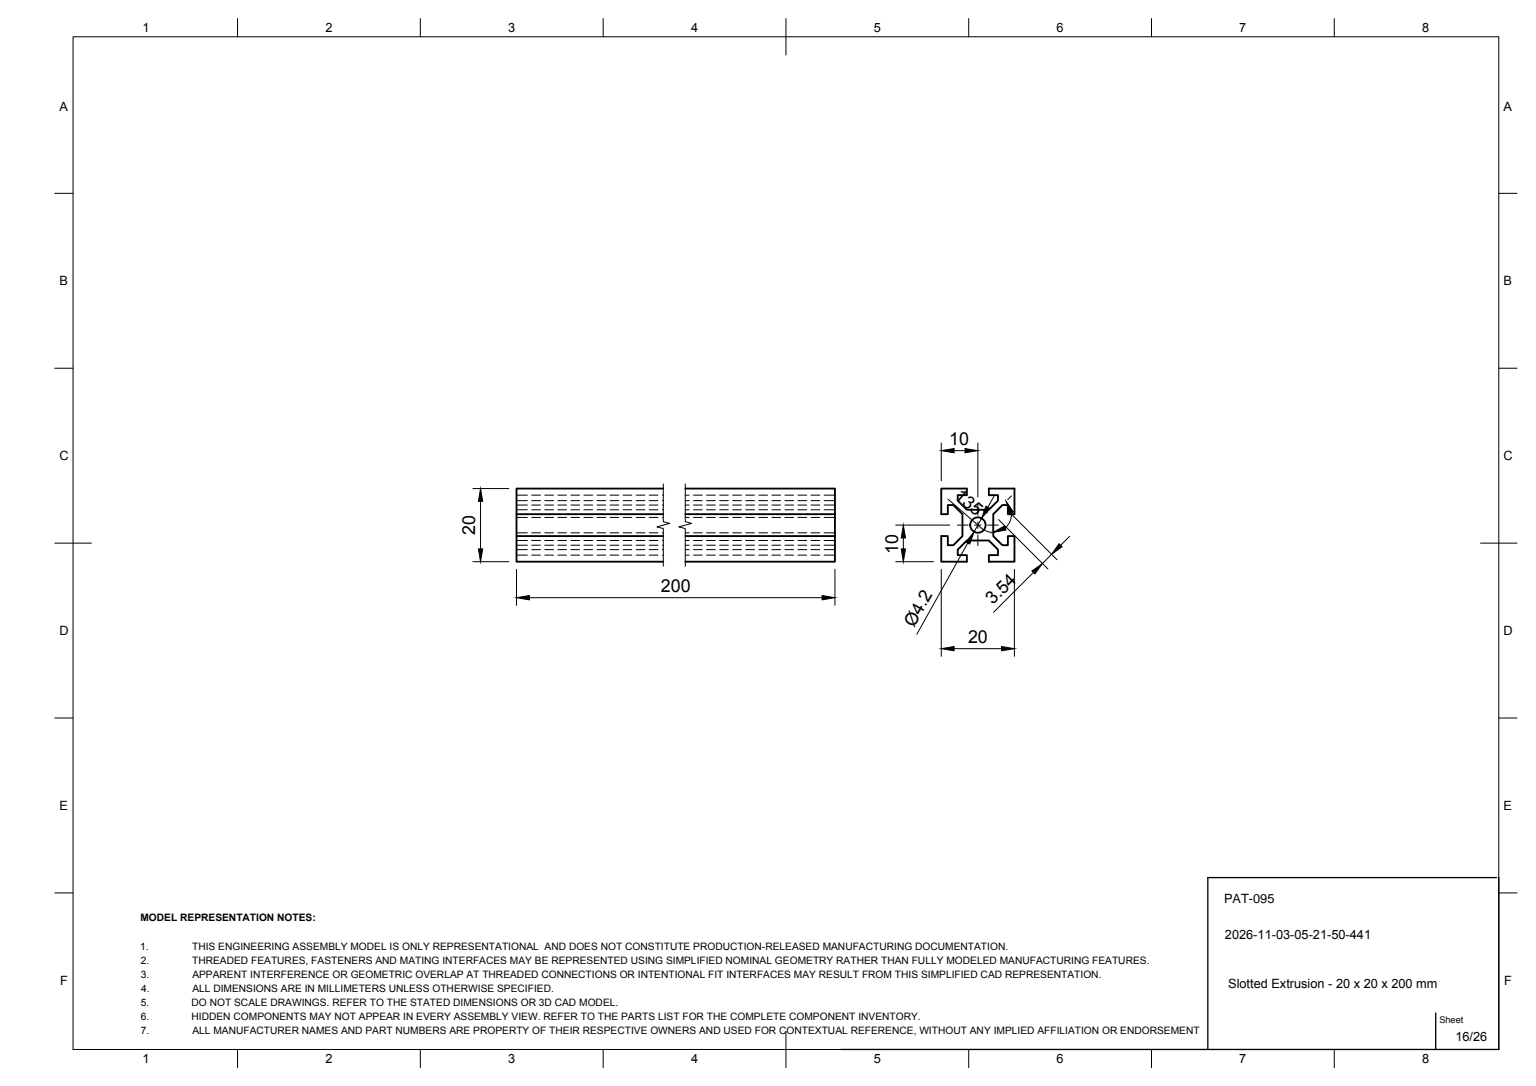
ISO-10303-21;
HEADER;
/* Generated by software containing ST-Developer
 * from STEP Tools, Inc. (www.steptools.com) 
 */

FILE_DESCRIPTION(
/* description */ ('Single-Axis Profile-Rail Linear Slide'),
/* implementation_level */ '2;1');

FILE_NAME(
/* name */ 'Slotted Extrusion - 20 x 20 x 200 mm.step',
/* time_stamp */ '2026-10-27T10:47:43-07:00',
/* author */ (''),
/* organization */ (''),
/* preprocessor_version */ 'ST-DEVELOPER v20.2',
/* originating_system */ 'Autodesk Translation Framework v15.17.0.0',
/* authorisation */ '');

FILE_SCHEMA (('AUTOMOTIVE_DESIGN { 1 0 10303 214 3 1 1 }'));
ENDSEC;

DATA;
#10=MECHANICAL_DESIGN_GEOMETRIC_PRESENTATION_REPRESENTATION('',(#340),#14478);
#286=SHAPE_REPRESENTATION_RELATIONSHIP('SRR','None',#14616,#313);
#313=ADVANCED_BREP_SHAPE_REPRESENTATION('',(#367),#14460);
#340=STYLED_ITEM('',(#14845),#367);
#367=MANIFOLD_SOLID_BREP('Body1',#8600);
#434=FACE_BOUND('',#1627,.T.);
#435=FACE_BOUND('',#1629,.T.);
#666=PLANE('',#9227);
#667=PLANE('',#9228);
#668=PLANE('',#9229);
#669=PLANE('',#9230);
#670=PLANE('',#9231);
#671=PLANE('',#9232);
#672=PLANE('',#9233);
#673=PLANE('',#9234);
#674=PLANE('',#9235);
#675=PLANE('',#9236);
#676=PLANE('',#9237);
#677=PLANE('',#9238);
#678=PLANE('',#9239);
#679=PLANE('',#9240);
#680=PLANE('',#9241);
#681=PLANE('',#9242);
#682=PLANE('',#9243);
#683=PLANE('',#9244);
#684=PLANE('',#9245);
#685=PLANE('',#9246);
#686=PLANE('',#9247);
#687=PLANE('',#9248);
#688=PLANE('',#9249);
#689=PLANE('',#9250);
#690=PLANE('',#9251);
#691=PLANE('',#9252);
#692=PLANE('',#9253);
#693=PLANE('',#9254);
#694=PLANE('',#9255);
#695=PLANE('',#9256);
#696=PLANE('',#9257);
#697=PLANE('',#9258);
#698=PLANE('',#9259);
#699=PLANE('',#9260);
#700=PLANE('',#9261);
#701=PLANE('',#9262);
#702=PLANE('',#9266);
#703=PLANE('',#9267);
#704=PLANE('',#9268);
#705=PLANE('',#9269);
#706=PLANE('',#9270);
#707=PLANE('',#9271);
#708=PLANE('',#9272);
#709=PLANE('',#9273);
#710=PLANE('',#9274);
#711=PLANE('',#9275);
#1070=FACE_OUTER_BOUND('',#1581,.T.);
#1071=FACE_OUTER_BOUND('',#1582,.T.);
#1072=FACE_OUTER_BOUND('',#1583,.T.);
#1073=FACE_OUTER_BOUND('',#1584,.T.);
#1074=FACE_OUTER_BOUND('',#1585,.T.);
#1075=FACE_OUTER_BOUND('',#1586,.T.);
#1076=FACE_OUTER_BOUND('',#1587,.T.);
#1077=FACE_OUTER_BOUND('',#1588,.T.);
#1078=FACE_OUTER_BOUND('',#1589,.T.);
#1079=FACE_OUTER_BOUND('',#1590,.T.);
#1080=FACE_OUTER_BOUND('',#1591,.T.);
#1081=FACE_OUTER_BOUND('',#1592,.T.);
#1082=FACE_OUTER_BOUND('',#1593,.T.);
#1083=FACE_OUTER_BOUND('',#1594,.T.);
#1084=FACE_OUTER_BOUND('',#1595,.T.);
#1085=FACE_OUTER_BOUND('',#1596,.T.);
#1086=FACE_OUTER_BOUND('',#1597,.T.);
#1087=FACE_OUTER_BOUND('',#1598,.T.);
#1088=FACE_OUTER_BOUND('',#1599,.T.);
#1089=FACE_OUTER_BOUND('',#1600,.T.);
#1090=FACE_OUTER_BOUND('',#1601,.T.);
#1091=FACE_OUTER_BOUND('',#1602,.T.);
#1092=FACE_OUTER_BOUND('',#1603,.T.);
#1093=FACE_OUTER_BOUND('',#1604,.T.);
#1094=FACE_OUTER_BOUND('',#1605,.T.);
#1095=FACE_OUTER_BOUND('',#1606,.T.);
#1096=FACE_OUTER_BOUND('',#1607,.T.);
#1097=FACE_OUTER_BOUND('',#1608,.T.);
#1098=FACE_OUTER_BOUND('',#1609,.T.);
#1099=FACE_OUTER_BOUND('',#1610,.T.);
#1100=FACE_OUTER_BOUND('',#1611,.T.);
#1101=FACE_OUTER_BOUND('',#1612,.T.);
#1102=FACE_OUTER_BOUND('',#1613,.T.);
#1103=FACE_OUTER_BOUND('',#1614,.T.);
#1104=FACE_OUTER_BOUND('',#1615,.T.);
#1105=FACE_OUTER_BOUND('',#1616,.T.);
#1106=FACE_OUTER_BOUND('',#1617,.T.);
#1107=FACE_OUTER_BOUND('',#1618,.T.);
#1108=FACE_OUTER_BOUND('',#1619,.T.);
#1109=FACE_OUTER_BOUND('',#1620,.T.);
#1110=FACE_OUTER_BOUND('',#1621,.T.);
#1111=FACE_OUTER_BOUND('',#1622,.T.);
#1112=FACE_OUTER_BOUND('',#1623,.T.);
#1113=FACE_OUTER_BOUND('',#1624,.T.);
#1114=FACE_OUTER_BOUND('',#1625,.T.);
#1115=FACE_OUTER_BOUND('',#1626,.T.);
#1116=FACE_OUTER_BOUND('',#1628,.T.);
#1581=EDGE_LOOP('',(#7013,#7014,#7015,#7016));
#1582=EDGE_LOOP('',(#7017,#7018,#7019,#7020));
#1583=EDGE_LOOP('',(#7021,#7022,#7023,#7024));
#1584=EDGE_LOOP('',(#7025,#7026,#7027,#7028));
#1585=EDGE_LOOP('',(#7029,#7030,#7031,#7032));
#1586=EDGE_LOOP('',(#7033,#7034,#7035,#7036));
#1587=EDGE_LOOP('',(#7037,#7038,#7039,#7040));
#1588=EDGE_LOOP('',(#7041,#7042,#7043,#7044));
#1589=EDGE_LOOP('',(#7045,#7046,#7047,#7048));
#1590=EDGE_LOOP('',(#7049,#7050,#7051,#7052));
#1591=EDGE_LOOP('',(#7053,#7054,#7055,#7056));
#1592=EDGE_LOOP('',(#7057,#7058,#7059,#7060));
#1593=EDGE_LOOP('',(#7061,#7062,#7063,#7064));
#1594=EDGE_LOOP('',(#7065,#7066,#7067,#7068));
#1595=EDGE_LOOP('',(#7069,#7070,#7071,#7072));
#1596=EDGE_LOOP('',(#7073,#7074,#7075,#7076));
#1597=EDGE_LOOP('',(#7077,#7078,#7079,#7080));
#1598=EDGE_LOOP('',(#7081,#7082,#7083,#7084));
#1599=EDGE_LOOP('',(#7085,#7086,#7087,#7088));
#1600=EDGE_LOOP('',(#7089,#7090,#7091,#7092));
#1601=EDGE_LOOP('',(#7093,#7094,#7095,#7096));
#1602=EDGE_LOOP('',(#7097,#7098,#7099,#7100));
#1603=EDGE_LOOP('',(#7101,#7102,#7103,#7104));
#1604=EDGE_LOOP('',(#7105,#7106,#7107,#7108));
#1605=EDGE_LOOP('',(#7109,#7110,#7111,#7112));
#1606=EDGE_LOOP('',(#7113,#7114,#7115,#7116));
#1607=EDGE_LOOP('',(#7117,#7118,#7119,#7120));
#1608=EDGE_LOOP('',(#7121,#7122,#7123,#7124));
#1609=EDGE_LOOP('',(#7125,#7126,#7127,#7128));
#1610=EDGE_LOOP('',(#7129,#7130,#7131,#7132));
#1611=EDGE_LOOP('',(#7133,#7134,#7135,#7136));
#1612=EDGE_LOOP('',(#7137,#7138,#7139,#7140));
#1613=EDGE_LOOP('',(#7141,#7142,#7143,#7144));
#1614=EDGE_LOOP('',(#7145,#7146,#7147,#7148));
#1615=EDGE_LOOP('',(#7149,#7150,#7151,#7152));
#1616=EDGE_LOOP('',(#7153,#7154,#7155,#7156));
#1617=EDGE_LOOP('',(#7157,#7158,#7159,#7160));
#1618=EDGE_LOOP('',(#7161,#7162,#7163,#7164));
#1619=EDGE_LOOP('',(#7165,#7166,#7167,#7168));
#1620=EDGE_LOOP('',(#7169,#7170,#7171,#7172));
#1621=EDGE_LOOP('',(#7173,#7174,#7175,#7176));
#1622=EDGE_LOOP('',(#7177,#7178,#7179,#7180));
#1623=EDGE_LOOP('',(#7181,#7182,#7183,#7184));
#1624=EDGE_LOOP('',(#7185,#7186,#7187,#7188));
#1625=EDGE_LOOP('',(#7189,#7190,#7191,#7192));
#1626=EDGE_LOOP('',(#7193,#7194,#7195,#7196,#7197,#7198,#7199,#7200,#7201,
#7202,#7203,#7204,#7205,#7206,#7207,#7208,#7209,#7210,#7211,#7212,#7213,
#7214,#7215,#7216,#7217,#7218,#7219,#7220,#7221,#7222,#7223,#7224,#7225,
#7226,#7227,#7228,#7229,#7230,#7231,#7232,#7233,#7234,#7235,#7236));
#1627=EDGE_LOOP('',(#7237));
#1628=EDGE_LOOP('',(#7238,#7239,#7240,#7241,#7242,#7243,#7244,#7245,#7246,
#7247,#7248,#7249,#7250,#7251,#7252,#7253,#7254,#7255,#7256,#7257,#7258,
#7259,#7260,#7261,#7262,#7263,#7264,#7265,#7266,#7267,#7268,#7269,#7270,
#7271,#7272,#7273,#7274,#7275,#7276,#7277,#7278,#7279,#7280,#7281));
#1629=EDGE_LOOP('',(#7282));
#2376=LINE('',#13243,#3347);
#2377=LINE('',#13245,#3348);
#2378=LINE('',#13247,#3349);
#2379=LINE('',#13248,#3350);
#2380=LINE('',#13251,#3351);
#2381=LINE('',#13253,#3352);
#2382=LINE('',#13254,#3353);
#2383=LINE('',#13257,#3354);
#2384=LINE('',#13259,#3355);
#2385=LINE('',#13260,#3356);
#2386=LINE('',#13263,#3357);
#2387=LINE('',#13265,#3358);
#2388=LINE('',#13266,#3359);
#2389=LINE('',#13269,#3360);
#2390=LINE('',#13271,#3361);
#2391=LINE('',#13272,#3362);
#2392=LINE('',#13275,#3363);
#2393=LINE('',#13277,#3364);
#2394=LINE('',#13278,#3365);
#2395=LINE('',#13281,#3366);
#2396=LINE('',#13283,#3367);
#2397=LINE('',#13284,#3368);
#2398=LINE('',#13287,#3369);
#2399=LINE('',#13289,#3370);
#2400=LINE('',#13290,#3371);
#2401=LINE('',#13293,#3372);
#2402=LINE('',#13295,#3373);
#2403=LINE('',#13296,#3374);
#2404=LINE('',#13300,#3375);
#2405=LINE('',#13302,#3376);
#2406=LINE('',#13304,#3377);
#2407=LINE('',#13305,#3378);
#2408=LINE('',#13308,#3379);
#2409=LINE('',#13310,#3380);
#2410=LINE('',#13311,#3381);
#2411=LINE('',#13314,#3382);
#2412=LINE('',#13316,#3383);
#2413=LINE('',#13317,#3384);
#2414=LINE('',#13320,#3385);
#2415=LINE('',#13322,#3386);
#2416=LINE('',#13323,#3387);
#2417=LINE('',#13326,#3388);
#2418=LINE('',#13328,#3389);
#2419=LINE('',#13329,#3390);
#2420=LINE('',#13332,#3391);
#2421=LINE('',#13334,#3392);
#2422=LINE('',#13335,#3393);
#2423=LINE('',#13338,#3394);
#2424=LINE('',#13340,#3395);
#2425=LINE('',#13341,#3396);
#2426=LINE('',#13344,#3397);
#2427=LINE('',#13346,#3398);
#2428=LINE('',#13347,#3399);
#2429=LINE('',#13350,#3400);
#2430=LINE('',#13352,#3401);
#2431=LINE('',#13353,#3402);
#2432=LINE('',#13357,#3403);
#2433=LINE('',#13359,#3404);
#2434=LINE('',#13361,#3405);
#2435=LINE('',#13362,#3406);
#2436=LINE('',#13365,#3407);
#2437=LINE('',#13367,#3408);
#2438=LINE('',#13368,#3409);
#2439=LINE('',#13371,#3410);
#2440=LINE('',#13373,#3411);
#2441=LINE('',#13374,#3412);
#2442=LINE('',#13377,#3413);
#2443=LINE('',#13379,#3414);
#2444=LINE('',#13380,#3415);
#2445=LINE('',#13383,#3416);
#2446=LINE('',#13385,#3417);
#2447=LINE('',#13386,#3418);
#2448=LINE('',#13389,#3419);
#2449=LINE('',#13391,#3420);
#2450=LINE('',#13392,#3421);
#2451=LINE('',#13395,#3422);
#2452=LINE('',#13397,#3423);
#2453=LINE('',#13398,#3424);
#2454=LINE('',#13401,#3425);
#2455=LINE('',#13403,#3426);
#2456=LINE('',#13404,#3427);
#2457=LINE('',#13407,#3428);
#2458=LINE('',#13409,#3429);
#2459=LINE('',#13410,#3430);
#2460=LINE('',#13414,#3431);
#2461=LINE('',#13416,#3432);
#2462=LINE('',#13418,#3433);
#2463=LINE('',#13419,#3434);
#2464=LINE('',#13422,#3435);
#2465=LINE('',#13424,#3436);
#2466=LINE('',#13425,#3437);
#2467=LINE('',#13428,#3438);
#2468=LINE('',#13430,#3439);
#2469=LINE('',#13431,#3440);
#2470=LINE('',#13434,#3441);
#2471=LINE('',#13436,#3442);
#2472=LINE('',#13437,#3443);
#2473=LINE('',#13440,#3444);
#2474=LINE('',#13442,#3445);
#2475=LINE('',#13443,#3446);
#2476=LINE('',#13446,#3447);
#2477=LINE('',#13448,#3448);
#2478=LINE('',#13449,#3449);
#2479=LINE('',#13452,#3450);
#2480=LINE('',#13454,#3451);
#2481=LINE('',#13455,#3452);
#2482=LINE('',#13458,#3453);
#2483=LINE('',#13460,#3454);
#2484=LINE('',#13461,#3455);
#2485=LINE('',#13464,#3456);
#2486=LINE('',#13466,#3457);
#2487=LINE('',#13467,#3458);
#2488=LINE('',#13472,#3459);
#2489=LINE('',#13476,#3460);
#2490=LINE('',#13478,#3461);
#2491=LINE('',#13479,#3462);
#2492=LINE('',#13482,#3463);
#2493=LINE('',#13484,#3464);
#2494=LINE('',#13485,#3465);
#2495=LINE('',#13487,#3466);
#2496=LINE('',#13488,#3467);
#2497=LINE('',#13491,#3468);
#2498=LINE('',#13493,#3469);
#2499=LINE('',#13494,#3470);
#2500=LINE('',#13496,#3471);
#2501=LINE('',#13497,#3472);
#2502=LINE('',#13500,#3473);
#2503=LINE('',#13502,#3474);
#2504=LINE('',#13503,#3475);
#2505=LINE('',#13505,#3476);
#2506=LINE('',#13506,#3477);
#2507=LINE('',#13508,#3478);
#2508=LINE('',#13509,#3479);
#3347=VECTOR('',#10775,1.);
#3348=VECTOR('',#10776,1.);
#3349=VECTOR('',#10777,1.);
#3350=VECTOR('',#10778,1.);
#3351=VECTOR('',#10781,1.);
#3352=VECTOR('',#10782,1.);
#3353=VECTOR('',#10783,1.);
#3354=VECTOR('',#10786,1.);
#3355=VECTOR('',#10787,1.);
#3356=VECTOR('',#10788,1.);
#3357=VECTOR('',#10791,1.);
#3358=VECTOR('',#10792,1.);
#3359=VECTOR('',#10793,1.);
#3360=VECTOR('',#10796,1.);
#3361=VECTOR('',#10797,1.);
#3362=VECTOR('',#10798,1.);
#3363=VECTOR('',#10801,1.);
#3364=VECTOR('',#10802,1.);
#3365=VECTOR('',#10803,1.);
#3366=VECTOR('',#10806,1.);
#3367=VECTOR('',#10807,1.);
#3368=VECTOR('',#10808,1.);
#3369=VECTOR('',#10811,1.);
#3370=VECTOR('',#10812,1.);
#3371=VECTOR('',#10813,1.);
#3372=VECTOR('',#10816,1.);
#3373=VECTOR('',#10817,1.);
#3374=VECTOR('',#10818,1.);
#3375=VECTOR('',#10821,1.);
#3376=VECTOR('',#10822,1.);
#3377=VECTOR('',#10823,1.);
#3378=VECTOR('',#10824,1.);
#3379=VECTOR('',#10827,1.);
#3380=VECTOR('',#10828,1.);
#3381=VECTOR('',#10829,1.);
#3382=VECTOR('',#10832,1.);
#3383=VECTOR('',#10833,1.);
#3384=VECTOR('',#10834,1.);
#3385=VECTOR('',#10837,1.);
#3386=VECTOR('',#10838,1.);
#3387=VECTOR('',#10839,1.);
#3388=VECTOR('',#10842,1.);
#3389=VECTOR('',#10843,1.);
#3390=VECTOR('',#10844,1.);
#3391=VECTOR('',#10847,1.);
#3392=VECTOR('',#10848,1.);
#3393=VECTOR('',#10849,1.);
#3394=VECTOR('',#10852,1.);
#3395=VECTOR('',#10853,1.);
#3396=VECTOR('',#10854,1.);
#3397=VECTOR('',#10857,1.);
#3398=VECTOR('',#10858,1.);
#3399=VECTOR('',#10859,1.);
#3400=VECTOR('',#10862,1.);
#3401=VECTOR('',#10863,1.);
#3402=VECTOR('',#10864,1.);
#3403=VECTOR('',#10867,1.);
#3404=VECTOR('',#10868,1.);
#3405=VECTOR('',#10869,1.);
#3406=VECTOR('',#10870,1.);
#3407=VECTOR('',#10873,1.);
#3408=VECTOR('',#10874,1.);
#3409=VECTOR('',#10875,1.);
#3410=VECTOR('',#10878,1.);
#3411=VECTOR('',#10879,1.);
#3412=VECTOR('',#10880,1.);
#3413=VECTOR('',#10883,1.);
#3414=VECTOR('',#10884,1.);
#3415=VECTOR('',#10885,1.);
#3416=VECTOR('',#10888,1.);
#3417=VECTOR('',#10889,1.);
#3418=VECTOR('',#10890,1.);
#3419=VECTOR('',#10893,1.);
#3420=VECTOR('',#10894,1.);
#3421=VECTOR('',#10895,1.);
#3422=VECTOR('',#10898,1.);
#3423=VECTOR('',#10899,1.);
#3424=VECTOR('',#10900,1.);
#3425=VECTOR('',#10903,1.);
#3426=VECTOR('',#10904,1.);
#3427=VECTOR('',#10905,1.);
#3428=VECTOR('',#10908,1.);
#3429=VECTOR('',#10909,1.);
#3430=VECTOR('',#10910,1.);
#3431=VECTOR('',#10913,1.);
#3432=VECTOR('',#10914,1.);
#3433=VECTOR('',#10915,1.);
#3434=VECTOR('',#10916,1.);
#3435=VECTOR('',#10919,1.);
#3436=VECTOR('',#10920,1.);
#3437=VECTOR('',#10921,1.);
#3438=VECTOR('',#10924,1.);
#3439=VECTOR('',#10925,1.);
#3440=VECTOR('',#10926,1.);
#3441=VECTOR('',#10929,1.);
#3442=VECTOR('',#10930,1.);
#3443=VECTOR('',#10931,1.);
#3444=VECTOR('',#10934,1.);
#3445=VECTOR('',#10935,1.);
#3446=VECTOR('',#10936,1.);
#3447=VECTOR('',#10939,1.);
#3448=VECTOR('',#10940,1.);
#3449=VECTOR('',#10941,1.);
#3450=VECTOR('',#10944,1.);
#3451=VECTOR('',#10945,1.);
#3452=VECTOR('',#10946,1.);
#3453=VECTOR('',#10949,1.);
#3454=VECTOR('',#10950,1.);
#3455=VECTOR('',#10951,1.);
#3456=VECTOR('',#10954,1.);
#3457=VECTOR('',#10955,1.);
#3458=VECTOR('',#10956,1.);
#3459=VECTOR('',#10961,0.21);
#3460=VECTOR('',#10966,1.);
#3461=VECTOR('',#10967,1.);
#3462=VECTOR('',#10968,1.);
#3463=VECTOR('',#10971,1.);
#3464=VECTOR('',#10972,1.);
#3465=VECTOR('',#10973,1.);
#3466=VECTOR('',#10976,1.);
#3467=VECTOR('',#10977,1.);
#3468=VECTOR('',#10980,1.);
#3469=VECTOR('',#10981,1.);
#3470=VECTOR('',#10982,1.);
#3471=VECTOR('',#10985,1.);
#3472=VECTOR('',#10986,1.);
#3473=VECTOR('',#10989,1.);
#3474=VECTOR('',#10990,1.);
#3475=VECTOR('',#10991,1.);
#3476=VECTOR('',#10994,1.);
#3477=VECTOR('',#10995,1.);
#3478=VECTOR('',#10998,1.);
#3479=VECTOR('',#10999,1.);
#3846=CIRCLE('',#9264,0.21);
#3847=CIRCLE('',#9265,0.21);
#4338=VERTEX_POINT('',#13241);
#4339=VERTEX_POINT('',#13242);
#4340=VERTEX_POINT('',#13244);
#4341=VERTEX_POINT('',#13246);
#4342=VERTEX_POINT('',#13250);
#4343=VERTEX_POINT('',#13252);
#4344=VERTEX_POINT('',#13256);
#4345=VERTEX_POINT('',#13258);
#4346=VERTEX_POINT('',#13262);
#4347=VERTEX_POINT('',#13264);
#4348=VERTEX_POINT('',#13268);
#4349=VERTEX_POINT('',#13270);
#4350=VERTEX_POINT('',#13274);
#4351=VERTEX_POINT('',#13276);
#4352=VERTEX_POINT('',#13280);
#4353=VERTEX_POINT('',#13282);
#4354=VERTEX_POINT('',#13286);
#4355=VERTEX_POINT('',#13288);
#4356=VERTEX_POINT('',#13292);
#4357=VERTEX_POINT('',#13294);
#4358=VERTEX_POINT('',#13298);
#4359=VERTEX_POINT('',#13299);
#4360=VERTEX_POINT('',#13301);
#4361=VERTEX_POINT('',#13303);
#4362=VERTEX_POINT('',#13307);
#4363=VERTEX_POINT('',#13309);
#4364=VERTEX_POINT('',#13313);
#4365=VERTEX_POINT('',#13315);
#4366=VERTEX_POINT('',#13319);
#4367=VERTEX_POINT('',#13321);
#4368=VERTEX_POINT('',#13325);
#4369=VERTEX_POINT('',#13327);
#4370=VERTEX_POINT('',#13331);
#4371=VERTEX_POINT('',#13333);
#4372=VERTEX_POINT('',#13337);
#4373=VERTEX_POINT('',#13339);
#4374=VERTEX_POINT('',#13343);
#4375=VERTEX_POINT('',#13345);
#4376=VERTEX_POINT('',#13349);
#4377=VERTEX_POINT('',#13351);
#4378=VERTEX_POINT('',#13355);
#4379=VERTEX_POINT('',#13356);
#4380=VERTEX_POINT('',#13358);
#4381=VERTEX_POINT('',#13360);
#4382=VERTEX_POINT('',#13364);
#4383=VERTEX_POINT('',#13366);
#4384=VERTEX_POINT('',#13370);
#4385=VERTEX_POINT('',#13372);
#4386=VERTEX_POINT('',#13376);
#4387=VERTEX_POINT('',#13378);
#4388=VERTEX_POINT('',#13382);
#4389=VERTEX_POINT('',#13384);
#4390=VERTEX_POINT('',#13388);
#4391=VERTEX_POINT('',#13390);
#4392=VERTEX_POINT('',#13394);
#4393=VERTEX_POINT('',#13396);
#4394=VERTEX_POINT('',#13400);
#4395=VERTEX_POINT('',#13402);
#4396=VERTEX_POINT('',#13406);
#4397=VERTEX_POINT('',#13408);
#4398=VERTEX_POINT('',#13412);
#4399=VERTEX_POINT('',#13413);
#4400=VERTEX_POINT('',#13415);
#4401=VERTEX_POINT('',#13417);
#4402=VERTEX_POINT('',#13421);
#4403=VERTEX_POINT('',#13423);
#4404=VERTEX_POINT('',#13427);
#4405=VERTEX_POINT('',#13429);
#4406=VERTEX_POINT('',#13433);
#4407=VERTEX_POINT('',#13435);
#4408=VERTEX_POINT('',#13439);
#4409=VERTEX_POINT('',#13441);
#4410=VERTEX_POINT('',#13445);
#4411=VERTEX_POINT('',#13447);
#4412=VERTEX_POINT('',#13451);
#4413=VERTEX_POINT('',#13453);
#4414=VERTEX_POINT('',#13457);
#4415=VERTEX_POINT('',#13459);
#4416=VERTEX_POINT('',#13463);
#4417=VERTEX_POINT('',#13465);
#4418=VERTEX_POINT('',#13469);
#4419=VERTEX_POINT('',#13471);
#4420=VERTEX_POINT('',#13475);
#4421=VERTEX_POINT('',#13477);
#4422=VERTEX_POINT('',#13481);
#4423=VERTEX_POINT('',#13483);
#4424=VERTEX_POINT('',#13490);
#4425=VERTEX_POINT('',#13492);
#4426=VERTEX_POINT('',#13499);
#4427=VERTEX_POINT('',#13501);
#5284=EDGE_CURVE('',#4338,#4339,#2376,.T.);
#5285=EDGE_CURVE('',#4338,#4340,#2377,.T.);
#5286=EDGE_CURVE('',#4341,#4340,#2378,.T.);
#5287=EDGE_CURVE('',#4339,#4341,#2379,.T.);
#5288=EDGE_CURVE('',#4342,#4338,#2380,.T.);
#5289=EDGE_CURVE('',#4342,#4343,#2381,.T.);
#5290=EDGE_CURVE('',#4340,#4343,#2382,.T.);
#5291=EDGE_CURVE('',#4344,#4342,#2383,.T.);
#5292=EDGE_CURVE('',#4344,#4345,#2384,.T.);
#5293=EDGE_CURVE('',#4343,#4345,#2385,.T.);
#5294=EDGE_CURVE('',#4346,#4344,#2386,.T.);
#5295=EDGE_CURVE('',#4346,#4347,#2387,.T.);
#5296=EDGE_CURVE('',#4345,#4347,#2388,.T.);
#5297=EDGE_CURVE('',#4348,#4346,#2389,.T.);
#5298=EDGE_CURVE('',#4348,#4349,#2390,.T.);
#5299=EDGE_CURVE('',#4347,#4349,#2391,.T.);
#5300=EDGE_CURVE('',#4350,#4348,#2392,.T.);
#5301=EDGE_CURVE('',#4350,#4351,#2393,.T.);
#5302=EDGE_CURVE('',#4349,#4351,#2394,.T.);
#5303=EDGE_CURVE('',#4352,#4350,#2395,.T.);
#5304=EDGE_CURVE('',#4352,#4353,#2396,.T.);
#5305=EDGE_CURVE('',#4351,#4353,#2397,.T.);
#5306=EDGE_CURVE('',#4354,#4352,#2398,.T.);
#5307=EDGE_CURVE('',#4354,#4355,#2399,.T.);
#5308=EDGE_CURVE('',#4353,#4355,#2400,.T.);
#5309=EDGE_CURVE('',#4356,#4354,#2401,.T.);
#5310=EDGE_CURVE('',#4357,#4356,#2402,.T.);
#5311=EDGE_CURVE('',#4355,#4357,#2403,.T.);
#5312=EDGE_CURVE('',#4358,#4359,#2404,.T.);
#5313=EDGE_CURVE('',#4358,#4360,#2405,.T.);
#5314=EDGE_CURVE('',#4361,#4360,#2406,.T.);
#5315=EDGE_CURVE('',#4359,#4361,#2407,.T.);
#5316=EDGE_CURVE('',#4362,#4358,#2408,.T.);
#5317=EDGE_CURVE('',#4362,#4363,#2409,.T.);
#5318=EDGE_CURVE('',#4360,#4363,#2410,.T.);
#5319=EDGE_CURVE('',#4364,#4362,#2411,.T.);
#5320=EDGE_CURVE('',#4364,#4365,#2412,.T.);
#5321=EDGE_CURVE('',#4363,#4365,#2413,.T.);
#5322=EDGE_CURVE('',#4366,#4364,#2414,.T.);
#5323=EDGE_CURVE('',#4366,#4367,#2415,.T.);
#5324=EDGE_CURVE('',#4365,#4367,#2416,.T.);
#5325=EDGE_CURVE('',#4368,#4366,#2417,.T.);
#5326=EDGE_CURVE('',#4368,#4369,#2418,.T.);
#5327=EDGE_CURVE('',#4367,#4369,#2419,.T.);
#5328=EDGE_CURVE('',#4370,#4368,#2420,.T.);
#5329=EDGE_CURVE('',#4370,#4371,#2421,.T.);
#5330=EDGE_CURVE('',#4369,#4371,#2422,.T.);
#5331=EDGE_CURVE('',#4372,#4370,#2423,.T.);
#5332=EDGE_CURVE('',#4372,#4373,#2424,.T.);
#5333=EDGE_CURVE('',#4371,#4373,#2425,.T.);
#5334=EDGE_CURVE('',#4374,#4372,#2426,.T.);
#5335=EDGE_CURVE('',#4374,#4375,#2427,.T.);
#5336=EDGE_CURVE('',#4373,#4375,#2428,.T.);
#5337=EDGE_CURVE('',#4376,#4374,#2429,.T.);
#5338=EDGE_CURVE('',#4377,#4376,#2430,.T.);
#5339=EDGE_CURVE('',#4375,#4377,#2431,.T.);
#5340=EDGE_CURVE('',#4378,#4379,#2432,.T.);
#5341=EDGE_CURVE('',#4378,#4380,#2433,.T.);
#5342=EDGE_CURVE('',#4381,#4380,#2434,.T.);
#5343=EDGE_CURVE('',#4379,#4381,#2435,.T.);
#5344=EDGE_CURVE('',#4382,#4378,#2436,.T.);
#5345=EDGE_CURVE('',#4382,#4383,#2437,.T.);
#5346=EDGE_CURVE('',#4380,#4383,#2438,.T.);
#5347=EDGE_CURVE('',#4384,#4382,#2439,.T.);
#5348=EDGE_CURVE('',#4384,#4385,#2440,.T.);
#5349=EDGE_CURVE('',#4383,#4385,#2441,.T.);
#5350=EDGE_CURVE('',#4386,#4384,#2442,.T.);
#5351=EDGE_CURVE('',#4386,#4387,#2443,.T.);
#5352=EDGE_CURVE('',#4385,#4387,#2444,.T.);
#5353=EDGE_CURVE('',#4388,#4386,#2445,.T.);
#5354=EDGE_CURVE('',#4388,#4389,#2446,.T.);
#5355=EDGE_CURVE('',#4387,#4389,#2447,.T.);
#5356=EDGE_CURVE('',#4390,#4388,#2448,.T.);
#5357=EDGE_CURVE('',#4390,#4391,#2449,.T.);
#5358=EDGE_CURVE('',#4389,#4391,#2450,.T.);
#5359=EDGE_CURVE('',#4392,#4390,#2451,.T.);
#5360=EDGE_CURVE('',#4392,#4393,#2452,.T.);
#5361=EDGE_CURVE('',#4391,#4393,#2453,.T.);
#5362=EDGE_CURVE('',#4394,#4392,#2454,.T.);
#5363=EDGE_CURVE('',#4394,#4395,#2455,.T.);
#5364=EDGE_CURVE('',#4393,#4395,#2456,.T.);
#5365=EDGE_CURVE('',#4396,#4394,#2457,.T.);
#5366=EDGE_CURVE('',#4397,#4396,#2458,.T.);
#5367=EDGE_CURVE('',#4395,#4397,#2459,.T.);
#5368=EDGE_CURVE('',#4398,#4399,#2460,.T.);
#5369=EDGE_CURVE('',#4398,#4400,#2461,.T.);
#5370=EDGE_CURVE('',#4401,#4400,#2462,.T.);
#5371=EDGE_CURVE('',#4399,#4401,#2463,.T.);
#5372=EDGE_CURVE('',#4402,#4398,#2464,.T.);
#5373=EDGE_CURVE('',#4402,#4403,#2465,.T.);
#5374=EDGE_CURVE('',#4400,#4403,#2466,.T.);
#5375=EDGE_CURVE('',#4404,#4402,#2467,.T.);
#5376=EDGE_CURVE('',#4404,#4405,#2468,.T.);
#5377=EDGE_CURVE('',#4403,#4405,#2469,.T.);
#5378=EDGE_CURVE('',#4406,#4404,#2470,.T.);
#5379=EDGE_CURVE('',#4406,#4407,#2471,.T.);
#5380=EDGE_CURVE('',#4405,#4407,#2472,.T.);
#5381=EDGE_CURVE('',#4408,#4406,#2473,.T.);
#5382=EDGE_CURVE('',#4408,#4409,#2474,.T.);
#5383=EDGE_CURVE('',#4407,#4409,#2475,.T.);
#5384=EDGE_CURVE('',#4410,#4408,#2476,.T.);
#5385=EDGE_CURVE('',#4410,#4411,#2477,.T.);
#5386=EDGE_CURVE('',#4409,#4411,#2478,.T.);
#5387=EDGE_CURVE('',#4412,#4410,#2479,.T.);
#5388=EDGE_CURVE('',#4412,#4413,#2480,.T.);
#5389=EDGE_CURVE('',#4411,#4413,#2481,.T.);
#5390=EDGE_CURVE('',#4414,#4412,#2482,.T.);
#5391=EDGE_CURVE('',#4414,#4415,#2483,.T.);
#5392=EDGE_CURVE('',#4413,#4415,#2484,.T.);
#5393=EDGE_CURVE('',#4416,#4414,#2485,.T.);
#5394=EDGE_CURVE('',#4417,#4416,#2486,.T.);
#5395=EDGE_CURVE('',#4415,#4417,#2487,.T.);
#5396=EDGE_CURVE('',#4418,#4418,#3846,.T.);
#5397=EDGE_CURVE('',#4418,#4419,#2488,.T.);
#5398=EDGE_CURVE('',#4419,#4419,#3847,.T.);
#5399=EDGE_CURVE('',#4356,#4420,#2489,.T.);
#5400=EDGE_CURVE('',#4420,#4421,#2490,.T.);
#5401=EDGE_CURVE('',#4357,#4421,#2491,.T.);
#5402=EDGE_CURVE('',#4422,#4341,#2492,.T.);
#5403=EDGE_CURVE('',#4423,#4422,#2493,.T.);
#5404=EDGE_CURVE('',#4423,#4339,#2494,.T.);
#5405=EDGE_CURVE('',#4376,#4423,#2495,.T.);
#5406=EDGE_CURVE('',#4377,#4422,#2496,.T.);
#5407=EDGE_CURVE('',#4424,#4361,#2497,.T.);
#5408=EDGE_CURVE('',#4425,#4424,#2498,.T.);
#5409=EDGE_CURVE('',#4425,#4359,#2499,.T.);
#5410=EDGE_CURVE('',#4396,#4425,#2500,.T.);
#5411=EDGE_CURVE('',#4397,#4424,#2501,.T.);
#5412=EDGE_CURVE('',#4426,#4381,#2502,.T.);
#5413=EDGE_CURVE('',#4427,#4426,#2503,.T.);
#5414=EDGE_CURVE('',#4427,#4379,#2504,.T.);
#5415=EDGE_CURVE('',#4416,#4427,#2505,.T.);
#5416=EDGE_CURVE('',#4417,#4426,#2506,.T.);
#5417=EDGE_CURVE('',#4421,#4401,#2507,.T.);
#5418=EDGE_CURVE('',#4420,#4399,#2508,.T.);
#7013=ORIENTED_EDGE('',*,*,#5284,.F.);
#7014=ORIENTED_EDGE('',*,*,#5285,.T.);
#7015=ORIENTED_EDGE('',*,*,#5286,.F.);
#7016=ORIENTED_EDGE('',*,*,#5287,.F.);
#7017=ORIENTED_EDGE('',*,*,#5288,.F.);
#7018=ORIENTED_EDGE('',*,*,#5289,.T.);
#7019=ORIENTED_EDGE('',*,*,#5290,.F.);
#7020=ORIENTED_EDGE('',*,*,#5285,.F.);
#7021=ORIENTED_EDGE('',*,*,#5291,.F.);
#7022=ORIENTED_EDGE('',*,*,#5292,.T.);
#7023=ORIENTED_EDGE('',*,*,#5293,.F.);
#7024=ORIENTED_EDGE('',*,*,#5289,.F.);
#7025=ORIENTED_EDGE('',*,*,#5294,.F.);
#7026=ORIENTED_EDGE('',*,*,#5295,.T.);
#7027=ORIENTED_EDGE('',*,*,#5296,.F.);
#7028=ORIENTED_EDGE('',*,*,#5292,.F.);
#7029=ORIENTED_EDGE('',*,*,#5297,.F.);
#7030=ORIENTED_EDGE('',*,*,#5298,.T.);
#7031=ORIENTED_EDGE('',*,*,#5299,.F.);
#7032=ORIENTED_EDGE('',*,*,#5295,.F.);
#7033=ORIENTED_EDGE('',*,*,#5300,.F.);
#7034=ORIENTED_EDGE('',*,*,#5301,.T.);
#7035=ORIENTED_EDGE('',*,*,#5302,.F.);
#7036=ORIENTED_EDGE('',*,*,#5298,.F.);
#7037=ORIENTED_EDGE('',*,*,#5303,.F.);
#7038=ORIENTED_EDGE('',*,*,#5304,.T.);
#7039=ORIENTED_EDGE('',*,*,#5305,.F.);
#7040=ORIENTED_EDGE('',*,*,#5301,.F.);
#7041=ORIENTED_EDGE('',*,*,#5306,.F.);
#7042=ORIENTED_EDGE('',*,*,#5307,.T.);
#7043=ORIENTED_EDGE('',*,*,#5308,.F.);
#7044=ORIENTED_EDGE('',*,*,#5304,.F.);
#7045=ORIENTED_EDGE('',*,*,#5309,.F.);
#7046=ORIENTED_EDGE('',*,*,#5310,.F.);
#7047=ORIENTED_EDGE('',*,*,#5311,.F.);
#7048=ORIENTED_EDGE('',*,*,#5307,.F.);
#7049=ORIENTED_EDGE('',*,*,#5312,.F.);
#7050=ORIENTED_EDGE('',*,*,#5313,.T.);
#7051=ORIENTED_EDGE('',*,*,#5314,.F.);
#7052=ORIENTED_EDGE('',*,*,#5315,.F.);
#7053=ORIENTED_EDGE('',*,*,#5316,.F.);
#7054=ORIENTED_EDGE('',*,*,#5317,.T.);
#7055=ORIENTED_EDGE('',*,*,#5318,.F.);
#7056=ORIENTED_EDGE('',*,*,#5313,.F.);
#7057=ORIENTED_EDGE('',*,*,#5319,.F.);
#7058=ORIENTED_EDGE('',*,*,#5320,.T.);
#7059=ORIENTED_EDGE('',*,*,#5321,.F.);
#7060=ORIENTED_EDGE('',*,*,#5317,.F.);
#7061=ORIENTED_EDGE('',*,*,#5322,.F.);
#7062=ORIENTED_EDGE('',*,*,#5323,.T.);
#7063=ORIENTED_EDGE('',*,*,#5324,.F.);
#7064=ORIENTED_EDGE('',*,*,#5320,.F.);
#7065=ORIENTED_EDGE('',*,*,#5325,.F.);
#7066=ORIENTED_EDGE('',*,*,#5326,.T.);
#7067=ORIENTED_EDGE('',*,*,#5327,.F.);
#7068=ORIENTED_EDGE('',*,*,#5323,.F.);
#7069=ORIENTED_EDGE('',*,*,#5328,.F.);
#7070=ORIENTED_EDGE('',*,*,#5329,.T.);
#7071=ORIENTED_EDGE('',*,*,#5330,.F.);
#7072=ORIENTED_EDGE('',*,*,#5326,.F.);
#7073=ORIENTED_EDGE('',*,*,#5331,.F.);
#7074=ORIENTED_EDGE('',*,*,#5332,.T.);
#7075=ORIENTED_EDGE('',*,*,#5333,.F.);
#7076=ORIENTED_EDGE('',*,*,#5329,.F.);
#7077=ORIENTED_EDGE('',*,*,#5334,.F.);
#7078=ORIENTED_EDGE('',*,*,#5335,.T.);
#7079=ORIENTED_EDGE('',*,*,#5336,.F.);
#7080=ORIENTED_EDGE('',*,*,#5332,.F.);
#7081=ORIENTED_EDGE('',*,*,#5337,.F.);
#7082=ORIENTED_EDGE('',*,*,#5338,.F.);
#7083=ORIENTED_EDGE('',*,*,#5339,.F.);
#7084=ORIENTED_EDGE('',*,*,#5335,.F.);
#7085=ORIENTED_EDGE('',*,*,#5340,.F.);
#7086=ORIENTED_EDGE('',*,*,#5341,.T.);
#7087=ORIENTED_EDGE('',*,*,#5342,.F.);
#7088=ORIENTED_EDGE('',*,*,#5343,.F.);
#7089=ORIENTED_EDGE('',*,*,#5344,.F.);
#7090=ORIENTED_EDGE('',*,*,#5345,.T.);
#7091=ORIENTED_EDGE('',*,*,#5346,.F.);
#7092=ORIENTED_EDGE('',*,*,#5341,.F.);
#7093=ORIENTED_EDGE('',*,*,#5347,.F.);
#7094=ORIENTED_EDGE('',*,*,#5348,.T.);
#7095=ORIENTED_EDGE('',*,*,#5349,.F.);
#7096=ORIENTED_EDGE('',*,*,#5345,.F.);
#7097=ORIENTED_EDGE('',*,*,#5350,.F.);
#7098=ORIENTED_EDGE('',*,*,#5351,.T.);
#7099=ORIENTED_EDGE('',*,*,#5352,.F.);
#7100=ORIENTED_EDGE('',*,*,#5348,.F.);
#7101=ORIENTED_EDGE('',*,*,#5353,.F.);
#7102=ORIENTED_EDGE('',*,*,#5354,.T.);
#7103=ORIENTED_EDGE('',*,*,#5355,.F.);
#7104=ORIENTED_EDGE('',*,*,#5351,.F.);
#7105=ORIENTED_EDGE('',*,*,#5356,.F.);
#7106=ORIENTED_EDGE('',*,*,#5357,.T.);
#7107=ORIENTED_EDGE('',*,*,#5358,.F.);
#7108=ORIENTED_EDGE('',*,*,#5354,.F.);
#7109=ORIENTED_EDGE('',*,*,#5359,.F.);
#7110=ORIENTED_EDGE('',*,*,#5360,.T.);
#7111=ORIENTED_EDGE('',*,*,#5361,.F.);
#7112=ORIENTED_EDGE('',*,*,#5357,.F.);
#7113=ORIENTED_EDGE('',*,*,#5362,.F.);
#7114=ORIENTED_EDGE('',*,*,#5363,.T.);
#7115=ORIENTED_EDGE('',*,*,#5364,.F.);
#7116=ORIENTED_EDGE('',*,*,#5360,.F.);
#7117=ORIENTED_EDGE('',*,*,#5365,.F.);
#7118=ORIENTED_EDGE('',*,*,#5366,.F.);
#7119=ORIENTED_EDGE('',*,*,#5367,.F.);
#7120=ORIENTED_EDGE('',*,*,#5363,.F.);
#7121=ORIENTED_EDGE('',*,*,#5368,.F.);
#7122=ORIENTED_EDGE('',*,*,#5369,.T.);
#7123=ORIENTED_EDGE('',*,*,#5370,.F.);
#7124=ORIENTED_EDGE('',*,*,#5371,.F.);
#7125=ORIENTED_EDGE('',*,*,#5372,.F.);
#7126=ORIENTED_EDGE('',*,*,#5373,.T.);
#7127=ORIENTED_EDGE('',*,*,#5374,.F.);
#7128=ORIENTED_EDGE('',*,*,#5369,.F.);
#7129=ORIENTED_EDGE('',*,*,#5375,.F.);
#7130=ORIENTED_EDGE('',*,*,#5376,.T.);
#7131=ORIENTED_EDGE('',*,*,#5377,.F.);
#7132=ORIENTED_EDGE('',*,*,#5373,.F.);
#7133=ORIENTED_EDGE('',*,*,#5378,.F.);
#7134=ORIENTED_EDGE('',*,*,#5379,.T.);
#7135=ORIENTED_EDGE('',*,*,#5380,.F.);
#7136=ORIENTED_EDGE('',*,*,#5376,.F.);
#7137=ORIENTED_EDGE('',*,*,#5381,.F.);
#7138=ORIENTED_EDGE('',*,*,#5382,.T.);
#7139=ORIENTED_EDGE('',*,*,#5383,.F.);
#7140=ORIENTED_EDGE('',*,*,#5379,.F.);
#7141=ORIENTED_EDGE('',*,*,#5384,.F.);
#7142=ORIENTED_EDGE('',*,*,#5385,.T.);
#7143=ORIENTED_EDGE('',*,*,#5386,.F.);
#7144=ORIENTED_EDGE('',*,*,#5382,.F.);
#7145=ORIENTED_EDGE('',*,*,#5387,.F.);
#7146=ORIENTED_EDGE('',*,*,#5388,.T.);
#7147=ORIENTED_EDGE('',*,*,#5389,.F.);
#7148=ORIENTED_EDGE('',*,*,#5385,.F.);
#7149=ORIENTED_EDGE('',*,*,#5390,.F.);
#7150=ORIENTED_EDGE('',*,*,#5391,.T.);
#7151=ORIENTED_EDGE('',*,*,#5392,.F.);
#7152=ORIENTED_EDGE('',*,*,#5388,.F.);
#7153=ORIENTED_EDGE('',*,*,#5393,.F.);
#7154=ORIENTED_EDGE('',*,*,#5394,.F.);
#7155=ORIENTED_EDGE('',*,*,#5395,.F.);
#7156=ORIENTED_EDGE('',*,*,#5391,.F.);
#7157=ORIENTED_EDGE('',*,*,#5396,.F.);
#7158=ORIENTED_EDGE('',*,*,#5397,.T.);
#7159=ORIENTED_EDGE('',*,*,#5398,.F.);
#7160=ORIENTED_EDGE('',*,*,#5397,.F.);
#7161=ORIENTED_EDGE('',*,*,#5310,.T.);
#7162=ORIENTED_EDGE('',*,*,#5399,.T.);
#7163=ORIENTED_EDGE('',*,*,#5400,.T.);
#7164=ORIENTED_EDGE('',*,*,#5401,.F.);
#7165=ORIENTED_EDGE('',*,*,#5287,.T.);
#7166=ORIENTED_EDGE('',*,*,#5402,.F.);
#7167=ORIENTED_EDGE('',*,*,#5403,.F.);
#7168=ORIENTED_EDGE('',*,*,#5404,.T.);
#7169=ORIENTED_EDGE('',*,*,#5338,.T.);
#7170=ORIENTED_EDGE('',*,*,#5405,.T.);
#7171=ORIENTED_EDGE('',*,*,#5403,.T.);
#7172=ORIENTED_EDGE('',*,*,#5406,.F.);
#7173=ORIENTED_EDGE('',*,*,#5315,.T.);
#7174=ORIENTED_EDGE('',*,*,#5407,.F.);
#7175=ORIENTED_EDGE('',*,*,#5408,.F.);
#7176=ORIENTED_EDGE('',*,*,#5409,.T.);
#7177=ORIENTED_EDGE('',*,*,#5366,.T.);
#7178=ORIENTED_EDGE('',*,*,#5410,.T.);
#7179=ORIENTED_EDGE('',*,*,#5408,.T.);
#7180=ORIENTED_EDGE('',*,*,#5411,.F.);
#7181=ORIENTED_EDGE('',*,*,#5343,.T.);
#7182=ORIENTED_EDGE('',*,*,#5412,.F.);
#7183=ORIENTED_EDGE('',*,*,#5413,.F.);
#7184=ORIENTED_EDGE('',*,*,#5414,.T.);
#7185=ORIENTED_EDGE('',*,*,#5394,.T.);
#7186=ORIENTED_EDGE('',*,*,#5415,.T.);
#7187=ORIENTED_EDGE('',*,*,#5413,.T.);
#7188=ORIENTED_EDGE('',*,*,#5416,.F.);
#7189=ORIENTED_EDGE('',*,*,#5371,.T.);
#7190=ORIENTED_EDGE('',*,*,#5417,.F.);
#7191=ORIENTED_EDGE('',*,*,#5400,.F.);
#7192=ORIENTED_EDGE('',*,*,#5418,.T.);
#7193=ORIENTED_EDGE('',*,*,#5286,.T.);
#7194=ORIENTED_EDGE('',*,*,#5290,.T.);
#7195=ORIENTED_EDGE('',*,*,#5293,.T.);
#7196=ORIENTED_EDGE('',*,*,#5296,.T.);
#7197=ORIENTED_EDGE('',*,*,#5299,.T.);
#7198=ORIENTED_EDGE('',*,*,#5302,.T.);
#7199=ORIENTED_EDGE('',*,*,#5305,.T.);
#7200=ORIENTED_EDGE('',*,*,#5308,.T.);
#7201=ORIENTED_EDGE('',*,*,#5311,.T.);
#7202=ORIENTED_EDGE('',*,*,#5401,.T.);
#7203=ORIENTED_EDGE('',*,*,#5417,.T.);
#7204=ORIENTED_EDGE('',*,*,#5370,.T.);
#7205=ORIENTED_EDGE('',*,*,#5374,.T.);
#7206=ORIENTED_EDGE('',*,*,#5377,.T.);
#7207=ORIENTED_EDGE('',*,*,#5380,.T.);
#7208=ORIENTED_EDGE('',*,*,#5383,.T.);
#7209=ORIENTED_EDGE('',*,*,#5386,.T.);
#7210=ORIENTED_EDGE('',*,*,#5389,.T.);
#7211=ORIENTED_EDGE('',*,*,#5392,.T.);
#7212=ORIENTED_EDGE('',*,*,#5395,.T.);
#7213=ORIENTED_EDGE('',*,*,#5416,.T.);
#7214=ORIENTED_EDGE('',*,*,#5412,.T.);
#7215=ORIENTED_EDGE('',*,*,#5342,.T.);
#7216=ORIENTED_EDGE('',*,*,#5346,.T.);
#7217=ORIENTED_EDGE('',*,*,#5349,.T.);
#7218=ORIENTED_EDGE('',*,*,#5352,.T.);
#7219=ORIENTED_EDGE('',*,*,#5355,.T.);
#7220=ORIENTED_EDGE('',*,*,#5358,.T.);
#7221=ORIENTED_EDGE('',*,*,#5361,.T.);
#7222=ORIENTED_EDGE('',*,*,#5364,.T.);
#7223=ORIENTED_EDGE('',*,*,#5367,.T.);
#7224=ORIENTED_EDGE('',*,*,#5411,.T.);
#7225=ORIENTED_EDGE('',*,*,#5407,.T.);
#7226=ORIENTED_EDGE('',*,*,#5314,.T.);
#7227=ORIENTED_EDGE('',*,*,#5318,.T.);
#7228=ORIENTED_EDGE('',*,*,#5321,.T.);
#7229=ORIENTED_EDGE('',*,*,#5324,.T.);
#7230=ORIENTED_EDGE('',*,*,#5327,.T.);
#7231=ORIENTED_EDGE('',*,*,#5330,.T.);
#7232=ORIENTED_EDGE('',*,*,#5333,.T.);
#7233=ORIENTED_EDGE('',*,*,#5336,.T.);
#7234=ORIENTED_EDGE('',*,*,#5339,.T.);
#7235=ORIENTED_EDGE('',*,*,#5406,.T.);
#7236=ORIENTED_EDGE('',*,*,#5402,.T.);
#7237=ORIENTED_EDGE('',*,*,#5398,.T.);
#7238=ORIENTED_EDGE('',*,*,#5284,.T.);
#7239=ORIENTED_EDGE('',*,*,#5404,.F.);
#7240=ORIENTED_EDGE('',*,*,#5405,.F.);
#7241=ORIENTED_EDGE('',*,*,#5337,.T.);
#7242=ORIENTED_EDGE('',*,*,#5334,.T.);
#7243=ORIENTED_EDGE('',*,*,#5331,.T.);
#7244=ORIENTED_EDGE('',*,*,#5328,.T.);
#7245=ORIENTED_EDGE('',*,*,#5325,.T.);
#7246=ORIENTED_EDGE('',*,*,#5322,.T.);
#7247=ORIENTED_EDGE('',*,*,#5319,.T.);
#7248=ORIENTED_EDGE('',*,*,#5316,.T.);
#7249=ORIENTED_EDGE('',*,*,#5312,.T.);
#7250=ORIENTED_EDGE('',*,*,#5409,.F.);
#7251=ORIENTED_EDGE('',*,*,#5410,.F.);
#7252=ORIENTED_EDGE('',*,*,#5365,.T.);
#7253=ORIENTED_EDGE('',*,*,#5362,.T.);
#7254=ORIENTED_EDGE('',*,*,#5359,.T.);
#7255=ORIENTED_EDGE('',*,*,#5356,.T.);
#7256=ORIENTED_EDGE('',*,*,#5353,.T.);
#7257=ORIENTED_EDGE('',*,*,#5350,.T.);
#7258=ORIENTED_EDGE('',*,*,#5347,.T.);
#7259=ORIENTED_EDGE('',*,*,#5344,.T.);
#7260=ORIENTED_EDGE('',*,*,#5340,.T.);
#7261=ORIENTED_EDGE('',*,*,#5414,.F.);
#7262=ORIENTED_EDGE('',*,*,#5415,.F.);
#7263=ORIENTED_EDGE('',*,*,#5393,.T.);
#7264=ORIENTED_EDGE('',*,*,#5390,.T.);
#7265=ORIENTED_EDGE('',*,*,#5387,.T.);
#7266=ORIENTED_EDGE('',*,*,#5384,.T.);
#7267=ORIENTED_EDGE('',*,*,#5381,.T.);
#7268=ORIENTED_EDGE('',*,*,#5378,.T.);
#7269=ORIENTED_EDGE('',*,*,#5375,.T.);
#7270=ORIENTED_EDGE('',*,*,#5372,.T.);
#7271=ORIENTED_EDGE('',*,*,#5368,.T.);
#7272=ORIENTED_EDGE('',*,*,#5418,.F.);
#7273=ORIENTED_EDGE('',*,*,#5399,.F.);
#7274=ORIENTED_EDGE('',*,*,#5309,.T.);
#7275=ORIENTED_EDGE('',*,*,#5306,.T.);
#7276=ORIENTED_EDGE('',*,*,#5303,.T.);
#7277=ORIENTED_EDGE('',*,*,#5300,.T.);
#7278=ORIENTED_EDGE('',*,*,#5297,.T.);
#7279=ORIENTED_EDGE('',*,*,#5294,.T.);
#7280=ORIENTED_EDGE('',*,*,#5291,.T.);
#7281=ORIENTED_EDGE('',*,*,#5288,.T.);
#7282=ORIENTED_EDGE('',*,*,#5396,.T.);
#8103=CYLINDRICAL_SURFACE('',#9263,0.21);
#8364=ADVANCED_FACE('',(#1070),#666,.F.);
#8365=ADVANCED_FACE('',(#1071),#667,.F.);
#8366=ADVANCED_FACE('',(#1072),#668,.F.);
#8367=ADVANCED_FACE('',(#1073),#669,.F.);
#8368=ADVANCED_FACE('',(#1074),#670,.F.);
#8369=ADVANCED_FACE('',(#1075),#671,.F.);
#8370=ADVANCED_FACE('',(#1076),#672,.F.);
#8371=ADVANCED_FACE('',(#1077),#673,.F.);
#8372=ADVANCED_FACE('',(#1078),#674,.F.);
#8373=ADVANCED_FACE('',(#1079),#675,.F.);
#8374=ADVANCED_FACE('',(#1080),#676,.F.);
#8375=ADVANCED_FACE('',(#1081),#677,.F.);
#8376=ADVANCED_FACE('',(#1082),#678,.F.);
#8377=ADVANCED_FACE('',(#1083),#679,.F.);
#8378=ADVANCED_FACE('',(#1084),#680,.F.);
#8379=ADVANCED_FACE('',(#1085),#681,.F.);
#8380=ADVANCED_FACE('',(#1086),#682,.F.);
#8381=ADVANCED_FACE('',(#1087),#683,.F.);
#8382=ADVANCED_FACE('',(#1088),#684,.F.);
#8383=ADVANCED_FACE('',(#1089),#685,.F.);
#8384=ADVANCED_FACE('',(#1090),#686,.F.);
#8385=ADVANCED_FACE('',(#1091),#687,.F.);
#8386=ADVANCED_FACE('',(#1092),#688,.F.);
#8387=ADVANCED_FACE('',(#1093),#689,.F.);
#8388=ADVANCED_FACE('',(#1094),#690,.F.);
#8389=ADVANCED_FACE('',(#1095),#691,.F.);
#8390=ADVANCED_FACE('',(#1096),#692,.F.);
#8391=ADVANCED_FACE('',(#1097),#693,.F.);
#8392=ADVANCED_FACE('',(#1098),#694,.F.);
#8393=ADVANCED_FACE('',(#1099),#695,.F.);
#8394=ADVANCED_FACE('',(#1100),#696,.F.);
#8395=ADVANCED_FACE('',(#1101),#697,.F.);
#8396=ADVANCED_FACE('',(#1102),#698,.F.);
#8397=ADVANCED_FACE('',(#1103),#699,.F.);
#8398=ADVANCED_FACE('',(#1104),#700,.F.);
#8399=ADVANCED_FACE('',(#1105),#701,.F.);
#8400=ADVANCED_FACE('',(#1106),#8103,.F.);
#8401=ADVANCED_FACE('',(#1107),#702,.T.);
#8402=ADVANCED_FACE('',(#1108),#703,.T.);
#8403=ADVANCED_FACE('',(#1109),#704,.T.);
#8404=ADVANCED_FACE('',(#1110),#705,.T.);
#8405=ADVANCED_FACE('',(#1111),#706,.T.);
#8406=ADVANCED_FACE('',(#1112),#707,.T.);
#8407=ADVANCED_FACE('',(#1113),#708,.T.);
#8408=ADVANCED_FACE('',(#1114),#709,.T.);
#8409=ADVANCED_FACE('',(#1115,#434),#710,.T.);
#8410=ADVANCED_FACE('',(#1116,#435),#711,.F.);
#8600=CLOSED_SHELL('',(#8364,#8365,#8366,#8367,#8368,#8369,#8370,#8371,
#8372,#8373,#8374,#8375,#8376,#8377,#8378,#8379,#8380,#8381,#8382,#8383,
#8384,#8385,#8386,#8387,#8388,#8389,#8390,#8391,#8392,#8393,#8394,#8395,
#8396,#8397,#8398,#8399,#8400,#8401,#8402,#8403,#8404,#8405,#8406,#8407,
#8408,#8409,#8410));
#9226=AXIS2_PLACEMENT_3D('',#13239,#10771,#10772);
#9227=AXIS2_PLACEMENT_3D('',#13240,#10773,#10774);
#9228=AXIS2_PLACEMENT_3D('',#13249,#10779,#10780);
#9229=AXIS2_PLACEMENT_3D('',#13255,#10784,#10785);
#9230=AXIS2_PLACEMENT_3D('',#13261,#10789,#10790);
#9231=AXIS2_PLACEMENT_3D('',#13267,#10794,#10795);
#9232=AXIS2_PLACEMENT_3D('',#13273,#10799,#10800);
#9233=AXIS2_PLACEMENT_3D('',#13279,#10804,#10805);
#9234=AXIS2_PLACEMENT_3D('',#13285,#10809,#10810);
#9235=AXIS2_PLACEMENT_3D('',#13291,#10814,#10815);
#9236=AXIS2_PLACEMENT_3D('',#13297,#10819,#10820);
#9237=AXIS2_PLACEMENT_3D('',#13306,#10825,#10826);
#9238=AXIS2_PLACEMENT_3D('',#13312,#10830,#10831);
#9239=AXIS2_PLACEMENT_3D('',#13318,#10835,#10836);
#9240=AXIS2_PLACEMENT_3D('',#13324,#10840,#10841);
#9241=AXIS2_PLACEMENT_3D('',#13330,#10845,#10846);
#9242=AXIS2_PLACEMENT_3D('',#13336,#10850,#10851);
#9243=AXIS2_PLACEMENT_3D('',#13342,#10855,#10856);
#9244=AXIS2_PLACEMENT_3D('',#13348,#10860,#10861);
#9245=AXIS2_PLACEMENT_3D('',#13354,#10865,#10866);
#9246=AXIS2_PLACEMENT_3D('',#13363,#10871,#10872);
#9247=AXIS2_PLACEMENT_3D('',#13369,#10876,#10877);
#9248=AXIS2_PLACEMENT_3D('',#13375,#10881,#10882);
#9249=AXIS2_PLACEMENT_3D('',#13381,#10886,#10887);
#9250=AXIS2_PLACEMENT_3D('',#13387,#10891,#10892);
#9251=AXIS2_PLACEMENT_3D('',#13393,#10896,#10897);
#9252=AXIS2_PLACEMENT_3D('',#13399,#10901,#10902);
#9253=AXIS2_PLACEMENT_3D('',#13405,#10906,#10907);
#9254=AXIS2_PLACEMENT_3D('',#13411,#10911,#10912);
#9255=AXIS2_PLACEMENT_3D('',#13420,#10917,#10918);
#9256=AXIS2_PLACEMENT_3D('',#13426,#10922,#10923);
#9257=AXIS2_PLACEMENT_3D('',#13432,#10927,#10928);
#9258=AXIS2_PLACEMENT_3D('',#13438,#10932,#10933);
#9259=AXIS2_PLACEMENT_3D('',#13444,#10937,#10938);
#9260=AXIS2_PLACEMENT_3D('',#13450,#10942,#10943);
#9261=AXIS2_PLACEMENT_3D('',#13456,#10947,#10948);
#9262=AXIS2_PLACEMENT_3D('',#13462,#10952,#10953);
#9263=AXIS2_PLACEMENT_3D('',#13468,#10957,#10958);
#9264=AXIS2_PLACEMENT_3D('',#13470,#10959,#10960);
#9265=AXIS2_PLACEMENT_3D('',#13473,#10962,#10963);
#9266=AXIS2_PLACEMENT_3D('',#13474,#10964,#10965);
#9267=AXIS2_PLACEMENT_3D('',#13480,#10969,#10970);
#9268=AXIS2_PLACEMENT_3D('',#13486,#10974,#10975);
#9269=AXIS2_PLACEMENT_3D('',#13489,#10978,#10979);
#9270=AXIS2_PLACEMENT_3D('',#13495,#10983,#10984);
#9271=AXIS2_PLACEMENT_3D('',#13498,#10987,#10988);
#9272=AXIS2_PLACEMENT_3D('',#13504,#10992,#10993);
#9273=AXIS2_PLACEMENT_3D('',#13507,#10996,#10997);
#9274=AXIS2_PLACEMENT_3D('',#13510,#11000,#11001);
#9275=AXIS2_PLACEMENT_3D('',#13511,#11002,#11003);
#10771=DIRECTION('axis',(0.,0.,1.));
#10772=DIRECTION('refdir',(1.,0.,0.));
#10773=DIRECTION('center_axis',(0.,0.,-1.));
#10774=DIRECTION('ref_axis',(0.,1.,0.));
#10775=DIRECTION('',(0.,1.,0.));
#10776=DIRECTION('',(1.,0.,0.));
#10777=DIRECTION('',(0.,-1.,0.));
#10778=DIRECTION('',(1.,0.,0.));
#10779=DIRECTION('center_axis',(0.,1.,-8.88178419700125E-16));
#10780=DIRECTION('ref_axis',(0.,8.88178419700125E-16,1.));
#10781=DIRECTION('',(0.,8.88178419700125E-16,1.));
#10782=DIRECTION('',(1.,0.,0.));
#10783=DIRECTION('',(0.,-8.88178419700125E-16,-1.));
#10784=DIRECTION('center_axis',(0.,-7.40148683083439E-16,-1.));
#10785=DIRECTION('ref_axis',(0.,1.,-7.40148683083439E-16));
#10786=DIRECTION('',(0.,1.,-7.40148683083439E-16));
#10787=DIRECTION('',(1.,0.,0.));
#10788=DIRECTION('',(0.,-1.,7.40148683083439E-16));
#10789=DIRECTION('center_axis',(0.,-0.707106781186547,-0.707106781186548));
#10790=DIRECTION('ref_axis',(0.,0.707106781186548,-0.707106781186547));
#10791=DIRECTION('',(0.,0.707106781186548,-0.707106781186547));
#10792=DIRECTION('',(1.,0.,0.));
#10793=DIRECTION('',(0.,-0.707106781186548,0.707106781186547));
#10794=DIRECTION('center_axis',(0.,-1.,2.77555756156289E-16));
#10795=DIRECTION('ref_axis',(0.,-2.77555756156289E-16,-1.));
#10796=DIRECTION('',(0.,-2.77555756156289E-16,-1.));
#10797=DIRECTION('',(1.,0.,0.));
#10798=DIRECTION('',(0.,2.77555756156289E-16,1.));
#10799=DIRECTION('center_axis',(0.,-0.707106781186547,0.707106781186548));
#10800=DIRECTION('ref_axis',(0.,-0.707106781186548,-0.707106781186547));
#10801=DIRECTION('',(0.,-0.707106781186548,-0.707106781186547));
#10802=DIRECTION('',(1.,0.,0.));
#10803=DIRECTION('',(0.,0.707106781186548,0.707106781186547));
#10804=DIRECTION('center_axis',(0.,7.40148683083438E-16,1.));
#10805=DIRECTION('ref_axis',(0.,-1.,7.40148683083438E-16));
#10806=DIRECTION('',(0.,-1.,7.40148683083438E-16));
#10807=DIRECTION('',(1.,0.,0.));
#10808=DIRECTION('',(0.,1.,-7.40148683083438E-16));
#10809=DIRECTION('center_axis',(0.,1.,-4.44089209850063E-16));
#10810=DIRECTION('ref_axis',(0.,4.44089209850063E-16,1.));
#10811=DIRECTION('',(0.,4.44089209850063E-16,1.));
#10812=DIRECTION('',(1.,0.,0.));
#10813=DIRECTION('',(0.,-4.44089209850063E-16,-1.));
#10814=DIRECTION('center_axis',(0.,2.41352831440251E-16,1.));
#10815=DIRECTION('ref_axis',(0.,-1.,2.41352831440251E-16));
#10816=DIRECTION('',(0.,-1.,2.41352831440251E-16));
#10817=DIRECTION('',(-1.,0.,0.));
#10818=DIRECTION('',(0.,1.,-2.41352831440251E-16));
#10819=DIRECTION('center_axis',(0.,-1.,2.41352831440251E-16));
#10820=DIRECTION('ref_axis',(0.,-2.41352831440251E-16,-1.));
#10821=DIRECTION('',(0.,-2.41352831440251E-16,-1.));
#10822=DIRECTION('',(1.,0.,0.));
#10823=DIRECTION('',(0.,2.41352831440251E-16,1.));
#10824=DIRECTION('',(1.,0.,0.));
#10825=DIRECTION('center_axis',(0.,0.,-1.));
#10826=DIRECTION('ref_axis',(0.,1.,0.));
#10827=DIRECTION('',(0.,1.,0.));
#10828=DIRECTION('',(1.,0.,0.));
#10829=DIRECTION('',(0.,-1.,0.));
#10830=DIRECTION('center_axis',(0.,-1.,0.));
#10831=DIRECTION('ref_axis',(0.,0.,-1.));
#10832=DIRECTION('',(0.,0.,-1.));
#10833=DIRECTION('',(1.,0.,0.));
#10834=DIRECTION('',(0.,0.,1.));
#10835=DIRECTION('center_axis',(0.,-0.707106781186547,0.707106781186548));
#10836=DIRECTION('ref_axis',(0.,-0.707106781186548,-0.707106781186547));
#10837=DIRECTION('',(0.,-0.707106781186548,-0.707106781186547));
#10838=DIRECTION('',(1.,0.,0.));
#10839=DIRECTION('',(0.,0.707106781186548,0.707106781186547));
#10840=DIRECTION('center_axis',(0.,0.,1.));
#10841=DIRECTION('ref_axis',(0.,-1.,0.));
#10842=DIRECTION('',(0.,-1.,0.));
#10843=DIRECTION('',(1.,0.,0.));
#10844=DIRECTION('',(0.,1.,0.));
#10845=DIRECTION('center_axis',(0.,0.707106781186548,0.707106781186547));
#10846=DIRECTION('ref_axis',(0.,-0.707106781186547,0.707106781186548));
#10847=DIRECTION('',(0.,-0.707106781186547,0.707106781186548));
#10848=DIRECTION('',(1.,0.,0.));
#10849=DIRECTION('',(0.,0.707106781186547,-0.707106781186548));
#10850=DIRECTION('center_axis',(0.,1.,0.));
#10851=DIRECTION('ref_axis',(0.,0.,1.));
#10852=DIRECTION('',(0.,0.,1.));
#10853=DIRECTION('',(1.,0.,0.));
#10854=DIRECTION('',(0.,0.,-1.));
#10855=DIRECTION('center_axis',(0.,0.,-1.));
#10856=DIRECTION('ref_axis',(0.,1.,0.));
#10857=DIRECTION('',(0.,1.,0.));
#10858=DIRECTION('',(1.,0.,0.));
#10859=DIRECTION('',(0.,-1.,0.));
#10860=DIRECTION('center_axis',(0.,1.,-2.41352831440251E-16));
#10861=DIRECTION('ref_axis',(0.,2.41352831440251E-16,1.));
#10862=DIRECTION('',(0.,2.41352831440251E-16,1.));
#10863=DIRECTION('',(-1.,0.,0.));
#10864=DIRECTION('',(0.,-2.41352831440251E-16,-1.));
#10865=DIRECTION('center_axis',(0.,0.,1.));
#10866=DIRECTION('ref_axis',(0.,-1.,0.));
#10867=DIRECTION('',(0.,-1.,0.));
#10868=DIRECTION('',(1.,0.,0.));
#10869=DIRECTION('',(0.,1.,0.));
#10870=DIRECTION('',(1.,0.,0.));
#10871=DIRECTION('center_axis',(0.,-1.,0.));
#10872=DIRECTION('ref_axis',(0.,0.,-1.));
#10873=DIRECTION('',(0.,0.,-1.));
#10874=DIRECTION('',(1.,0.,0.));
#10875=DIRECTION('',(0.,0.,1.));
#10876=DIRECTION('center_axis',(0.,0.,1.));
#10877=DIRECTION('ref_axis',(0.,-1.,0.));
#10878=DIRECTION('',(0.,-1.,0.));
#10879=DIRECTION('',(1.,0.,0.));
#10880=DIRECTION('',(0.,1.,0.));
#10881=DIRECTION('center_axis',(0.,0.707106781186548,0.707106781186548));
#10882=DIRECTION('ref_axis',(0.,-0.707106781186548,0.707106781186548));
#10883=DIRECTION('',(0.,-0.707106781186548,0.707106781186548));
#10884=DIRECTION('',(1.,0.,0.));
#10885=DIRECTION('',(0.,0.707106781186548,-0.707106781186548));
#10886=DIRECTION('center_axis',(0.,1.,0.));
#10887=DIRECTION('ref_axis',(0.,0.,1.));
#10888=DIRECTION('',(0.,0.,1.));
#10889=DIRECTION('',(1.,0.,0.));
#10890=DIRECTION('',(0.,0.,-1.));
#10891=DIRECTION('center_axis',(0.,0.707106781186548,-0.707106781186547));
#10892=DIRECTION('ref_axis',(0.,0.707106781186547,0.707106781186548));
#10893=DIRECTION('',(0.,0.707106781186547,0.707106781186548));
#10894=DIRECTION('',(1.,0.,0.));
#10895=DIRECTION('',(0.,-0.707106781186547,-0.707106781186548));
#10896=DIRECTION('center_axis',(0.,-7.40148683083438E-16,-1.));
#10897=DIRECTION('ref_axis',(0.,1.,-7.40148683083438E-16));
#10898=DIRECTION('',(0.,1.,-7.40148683083438E-16));
#10899=DIRECTION('',(1.,0.,0.));
#10900=DIRECTION('',(0.,-1.,7.40148683083438E-16));
#10901=DIRECTION('center_axis',(0.,-1.,0.));
#10902=DIRECTION('ref_axis',(0.,0.,-1.));
#10903=DIRECTION('',(0.,0.,-1.));
#10904=DIRECTION('',(1.,0.,0.));
#10905=DIRECTION('',(0.,0.,1.));
#10906=DIRECTION('center_axis',(0.,0.,-1.));
#10907=DIRECTION('ref_axis',(0.,1.,0.));
#10908=DIRECTION('',(0.,1.,0.));
#10909=DIRECTION('',(-1.,0.,0.));
#10910=DIRECTION('',(0.,-1.,0.));
#10911=DIRECTION('center_axis',(0.,1.,0.));
#10912=DIRECTION('ref_axis',(0.,0.,1.));
#10913=DIRECTION('',(0.,0.,1.));
#10914=DIRECTION('',(1.,0.,0.));
#10915=DIRECTION('',(0.,0.,-1.));
#10916=DIRECTION('',(1.,0.,0.));
#10917=DIRECTION('center_axis',(0.,0.,1.));
#10918=DIRECTION('ref_axis',(0.,-1.,0.));
#10919=DIRECTION('',(0.,-1.,0.));
#10920=DIRECTION('',(1.,0.,0.));
#10921=DIRECTION('',(0.,1.,0.));
#10922=DIRECTION('center_axis',(0.,1.,0.));
#10923=DIRECTION('ref_axis',(0.,0.,1.));
#10924=DIRECTION('',(0.,0.,1.));
#10925=DIRECTION('',(1.,0.,0.));
#10926=DIRECTION('',(0.,0.,-1.));
#10927=DIRECTION('center_axis',(0.,0.707106781186547,-0.707106781186548));
#10928=DIRECTION('ref_axis',(0.,0.707106781186548,0.707106781186547));
#10929=DIRECTION('',(0.,0.707106781186548,0.707106781186547));
#10930=DIRECTION('',(1.,0.,0.));
#10931=DIRECTION('',(0.,-0.707106781186548,-0.707106781186547));
#10932=DIRECTION('center_axis',(0.,0.,-1.));
#10933=DIRECTION('ref_axis',(0.,1.,0.));
#10934=DIRECTION('',(0.,1.,0.));
#10935=DIRECTION('',(1.,0.,0.));
#10936=DIRECTION('',(0.,-1.,0.));
#10937=DIRECTION('center_axis',(0.,-0.707106781186547,-0.707106781186548));
#10938=DIRECTION('ref_axis',(0.,0.707106781186548,-0.707106781186547));
#10939=DIRECTION('',(0.,0.707106781186548,-0.707106781186547));
#10940=DIRECTION('',(1.,0.,0.));
#10941=DIRECTION('',(0.,-0.707106781186548,0.707106781186547));
#10942=DIRECTION('center_axis',(0.,-1.,0.));
#10943=DIRECTION('ref_axis',(0.,0.,-1.));
#10944=DIRECTION('',(0.,0.,-1.));
#10945=DIRECTION('',(1.,0.,0.));
#10946=DIRECTION('',(0.,0.,1.));
#10947=DIRECTION('center_axis',(0.,0.,1.));
#10948=DIRECTION('ref_axis',(0.,-1.,0.));
#10949=DIRECTION('',(0.,-1.,0.));
#10950=DIRECTION('',(1.,0.,0.));
#10951=DIRECTION('',(0.,1.,0.));
#10952=DIRECTION('center_axis',(0.,-1.,0.));
#10953=DIRECTION('ref_axis',(0.,0.,-1.));
#10954=DIRECTION('',(0.,0.,-1.));
#10955=DIRECTION('',(-1.,0.,0.));
#10956=DIRECTION('',(0.,0.,1.));
#10957=DIRECTION('center_axis',(1.,0.,0.));
#10958=DIRECTION('ref_axis',(0.,0.,-1.));
#10959=DIRECTION('center_axis',(1.,0.,0.));
#10960=DIRECTION('ref_axis',(0.,0.,-1.));
#10961=DIRECTION('',(1.,0.,0.));
#10962=DIRECTION('center_axis',(-1.,0.,0.));
#10963=DIRECTION('ref_axis',(0.,0.,-1.));
#10964=DIRECTION('center_axis',(0.,1.,0.));
#10965=DIRECTION('ref_axis',(0.,0.,1.));
#10966=DIRECTION('',(0.,0.,1.));
#10967=DIRECTION('',(1.,0.,0.));
#10968=DIRECTION('',(0.,0.,1.));
#10969=DIRECTION('center_axis',(0.,1.,0.));
#10970=DIRECTION('ref_axis',(0.,0.,1.));
#10971=DIRECTION('',(0.,0.,1.));
#10972=DIRECTION('',(1.,0.,0.));
#10973=DIRECTION('',(0.,0.,1.));
#10974=DIRECTION('center_axis',(0.,0.,-1.));
#10975=DIRECTION('ref_axis',(0.,1.,0.));
#10976=DIRECTION('',(0.,1.,0.));
#10977=DIRECTION('',(0.,1.,0.));
#10978=DIRECTION('center_axis',(0.,0.,-1.));
#10979=DIRECTION('ref_axis',(0.,1.,0.));
#10980=DIRECTION('',(0.,1.,0.));
#10981=DIRECTION('',(1.,0.,0.));
#10982=DIRECTION('',(0.,1.,0.));
#10983=DIRECTION('center_axis',(0.,-1.,0.));
#10984=DIRECTION('ref_axis',(0.,0.,-1.));
#10985=DIRECTION('',(0.,0.,-1.));
#10986=DIRECTION('',(0.,0.,-1.));
#10987=DIRECTION('center_axis',(0.,-1.,0.));
#10988=DIRECTION('ref_axis',(0.,0.,-1.));
#10989=DIRECTION('',(0.,0.,-1.));
#10990=DIRECTION('',(1.,0.,0.));
#10991=DIRECTION('',(0.,0.,-1.));
#10992=DIRECTION('center_axis',(0.,0.,1.));
#10993=DIRECTION('ref_axis',(0.,-1.,0.));
#10994=DIRECTION('',(0.,-1.,0.));
#10995=DIRECTION('',(0.,-1.,0.));
#10996=DIRECTION('center_axis',(0.,0.,1.));
#10997=DIRECTION('ref_axis',(0.,-1.,0.));
#10998=DIRECTION('',(0.,-1.,0.));
#10999=DIRECTION('',(0.,-1.,0.));
#11000=DIRECTION('center_axis',(1.,0.,0.));
#11001=DIRECTION('ref_axis',(0.,0.,-1.));
#11002=DIRECTION('center_axis',(1.,0.,0.));
#11003=DIRECTION('ref_axis',(0.,0.,-1.));
#13239=CARTESIAN_POINT('',(0.,0.,0.));
#13240=CARTESIAN_POINT('Origin',(-0.1,0.82,-0.3));
#13241=CARTESIAN_POINT('',(0.,0.82,-0.3));
#13242=CARTESIAN_POINT('',(0.,1.,-0.3));
#13243=CARTESIAN_POINT('',(0.,0.41,-0.3));
#13244=CARTESIAN_POINT('',(20.,0.82,-0.3));
#13245=CARTESIAN_POINT('',(-0.1,0.82,-0.3));
#13246=CARTESIAN_POINT('',(20.,1.,-0.3));
#13247=CARTESIAN_POINT('',(20.,0.41,-0.3));
#13248=CARTESIAN_POINT('',(-0.05,1.,-0.3));
#13249=CARTESIAN_POINT('Origin',(-0.1,0.82,-0.55));
#13250=CARTESIAN_POINT('',(0.,0.82,-0.55));
#13251=CARTESIAN_POINT('',(0.,0.82,-0.275));
#13252=CARTESIAN_POINT('',(20.,0.82,-0.55));
#13253=CARTESIAN_POINT('',(-0.1,0.82,-0.55));
#13254=CARTESIAN_POINT('',(20.,0.82,-0.275));
#13255=CARTESIAN_POINT('Origin',(-0.1,0.67,-0.55));
#13256=CARTESIAN_POINT('',(0.,0.67,-0.55));
#13257=CARTESIAN_POINT('',(0.,0.335,-0.55));
#13258=CARTESIAN_POINT('',(20.,0.67,-0.55));
#13259=CARTESIAN_POINT('',(-0.1,0.67,-0.55));
#13260=CARTESIAN_POINT('',(20.,0.335,-0.55));
#13261=CARTESIAN_POINT('Origin',(-0.1,0.42,-0.3));
#13262=CARTESIAN_POINT('',(0.,0.42,-0.3));
#13263=CARTESIAN_POINT('',(0.,0.24,-0.12));
#13264=CARTESIAN_POINT('',(20.,0.42,-0.3));
#13265=CARTESIAN_POINT('',(-0.1,0.42,-0.3));
#13266=CARTESIAN_POINT('',(20.,0.24,-0.12));
#13267=CARTESIAN_POINT('Origin',(-0.1,0.42,0.3));
#13268=CARTESIAN_POINT('',(0.,0.42,0.3));
#13269=CARTESIAN_POINT('',(0.,0.42,0.15));
#13270=CARTESIAN_POINT('',(20.,0.42,0.3));
#13271=CARTESIAN_POINT('',(-0.1,0.42,0.3));
#13272=CARTESIAN_POINT('',(20.,0.42,0.15));
#13273=CARTESIAN_POINT('Origin',(-0.1,0.67,0.55));
#13274=CARTESIAN_POINT('',(0.,0.67,0.55));
#13275=CARTESIAN_POINT('',(6.93889390390723E-18,0.365,0.245));
#13276=CARTESIAN_POINT('',(20.,0.67,0.55));
#13277=CARTESIAN_POINT('',(-0.1,0.67,0.55));
#13278=CARTESIAN_POINT('',(20.,0.365,0.245));
#13279=CARTESIAN_POINT('Origin',(-0.1,0.82,0.55));
#13280=CARTESIAN_POINT('',(0.,0.82,0.55));
#13281=CARTESIAN_POINT('',(0.,0.41,0.55));
#13282=CARTESIAN_POINT('',(20.,0.82,0.55));
#13283=CARTESIAN_POINT('',(-0.1,0.82,0.55));
#13284=CARTESIAN_POINT('',(20.,0.41,0.55));
#13285=CARTESIAN_POINT('Origin',(-0.1,0.82,0.3));
#13286=CARTESIAN_POINT('',(0.,0.82,0.3));
#13287=CARTESIAN_POINT('',(0.,0.82,0.15));
#13288=CARTESIAN_POINT('',(20.,0.82,0.3));
#13289=CARTESIAN_POINT('',(-0.1,0.82,0.3));
#13290=CARTESIAN_POINT('',(20.,0.82,0.15));
#13291=CARTESIAN_POINT('Origin',(-0.1,1.05,0.3));
#13292=CARTESIAN_POINT('',(0.,1.,0.3));
#13293=CARTESIAN_POINT('',(0.,0.525,0.3));
#13294=CARTESIAN_POINT('',(20.,1.,0.3));
#13295=CARTESIAN_POINT('',(-0.05,1.,0.3));
#13296=CARTESIAN_POINT('',(20.,0.525,0.3));
#13297=CARTESIAN_POINT('Origin',(-0.1,-0.3,-0.82));
#13298=CARTESIAN_POINT('',(0.,-0.3,-0.82));
#13299=CARTESIAN_POINT('',(0.,-0.3,-1.));
#13300=CARTESIAN_POINT('',(0.,-0.3,-0.41));
#13301=CARTESIAN_POINT('',(20.,-0.3,-0.82));
#13302=CARTESIAN_POINT('',(-0.1,-0.3,-0.82));
#13303=CARTESIAN_POINT('',(20.,-0.3,-1.));
#13304=CARTESIAN_POINT('',(20.,-0.3,-0.41));
#13305=CARTESIAN_POINT('',(-0.05,-0.3,-1.));
#13306=CARTESIAN_POINT('Origin',(-0.1,-0.55,-0.82));
#13307=CARTESIAN_POINT('',(0.,-0.55,-0.82));
#13308=CARTESIAN_POINT('',(0.,-0.275,-0.82));
#13309=CARTESIAN_POINT('',(20.,-0.55,-0.82));
#13310=CARTESIAN_POINT('',(-0.1,-0.55,-0.82));
#13311=CARTESIAN_POINT('',(20.,-0.275,-0.82));
#13312=CARTESIAN_POINT('Origin',(-0.1,-0.55,-0.67));
#13313=CARTESIAN_POINT('',(0.,-0.55,-0.67));
#13314=CARTESIAN_POINT('',(0.,-0.55,-0.335));
#13315=CARTESIAN_POINT('',(20.,-0.55,-0.67));
#13316=CARTESIAN_POINT('',(-0.1,-0.55,-0.67));
#13317=CARTESIAN_POINT('',(20.,-0.55,-0.335));
#13318=CARTESIAN_POINT('Origin',(-0.1,-0.3,-0.42));
#13319=CARTESIAN_POINT('',(0.,-0.3,-0.42));
#13320=CARTESIAN_POINT('',(0.,-0.12,-0.24));
#13321=CARTESIAN_POINT('',(20.,-0.3,-0.42));
#13322=CARTESIAN_POINT('',(-0.1,-0.3,-0.42));
#13323=CARTESIAN_POINT('',(20.,-0.12,-0.24));
#13324=CARTESIAN_POINT('Origin',(-0.1,0.3,-0.42));
#13325=CARTESIAN_POINT('',(0.,0.3,-0.42));
#13326=CARTESIAN_POINT('',(0.,0.15,-0.42));
#13327=CARTESIAN_POINT('',(20.,0.3,-0.42));
#13328=CARTESIAN_POINT('',(-0.1,0.3,-0.42));
#13329=CARTESIAN_POINT('',(20.,0.15,-0.42));
#13330=CARTESIAN_POINT('Origin',(-0.1,0.55,-0.67));
#13331=CARTESIAN_POINT('',(0.,0.55,-0.67));
#13332=CARTESIAN_POINT('',(0.,0.245,-0.365));
#13333=CARTESIAN_POINT('',(20.,0.55,-0.67));
#13334=CARTESIAN_POINT('',(-0.1,0.55,-0.67));
#13335=CARTESIAN_POINT('',(20.,0.245,-0.365));
#13336=CARTESIAN_POINT('Origin',(-0.1,0.55,-0.82));
#13337=CARTESIAN_POINT('',(0.,0.55,-0.82));
#13338=CARTESIAN_POINT('',(0.,0.55,-0.41));
#13339=CARTESIAN_POINT('',(20.,0.55,-0.82));
#13340=CARTESIAN_POINT('',(-0.1,0.55,-0.82));
#13341=CARTESIAN_POINT('',(20.,0.55,-0.41));
#13342=CARTESIAN_POINT('Origin',(-0.1,0.3,-0.82));
#13343=CARTESIAN_POINT('',(0.,0.3,-0.82));
#13344=CARTESIAN_POINT('',(0.,0.15,-0.82));
#13345=CARTESIAN_POINT('',(20.,0.3,-0.82));
#13346=CARTESIAN_POINT('',(-0.1,0.3,-0.82));
#13347=CARTESIAN_POINT('',(20.,0.15,-0.82));
#13348=CARTESIAN_POINT('Origin',(-0.1,0.3,-1.05));
#13349=CARTESIAN_POINT('',(0.,0.3,-1.));
#13350=CARTESIAN_POINT('',(0.,0.3,-0.525));
#13351=CARTESIAN_POINT('',(20.,0.3,-1.));
#13352=CARTESIAN_POINT('',(-0.05,0.3,-1.));
#13353=CARTESIAN_POINT('',(20.,0.3,-0.525));
#13354=CARTESIAN_POINT('Origin',(-0.1,-0.82,0.3));
#13355=CARTESIAN_POINT('',(0.,-0.82,0.3));
#13356=CARTESIAN_POINT('',(0.,-1.,0.3));
#13357=CARTESIAN_POINT('',(0.,-0.41,0.3));
#13358=CARTESIAN_POINT('',(20.,-0.82,0.3));
#13359=CARTESIAN_POINT('',(-0.1,-0.82,0.3));
#13360=CARTESIAN_POINT('',(20.,-1.,0.3));
#13361=CARTESIAN_POINT('',(20.,-0.41,0.3));
#13362=CARTESIAN_POINT('',(-0.05,-1.,0.3));
#13363=CARTESIAN_POINT('Origin',(-0.1,-0.82,0.55));
#13364=CARTESIAN_POINT('',(0.,-0.82,0.55));
#13365=CARTESIAN_POINT('',(0.,-0.82,0.275));
#13366=CARTESIAN_POINT('',(20.,-0.82,0.55));
#13367=CARTESIAN_POINT('',(-0.1,-0.82,0.55));
#13368=CARTESIAN_POINT('',(20.,-0.82,0.275));
#13369=CARTESIAN_POINT('Origin',(-0.1,-0.67,0.55));
#13370=CARTESIAN_POINT('',(0.,-0.67,0.55));
#13371=CARTESIAN_POINT('',(0.,-0.335,0.55));
#13372=CARTESIAN_POINT('',(20.,-0.67,0.55));
#13373=CARTESIAN_POINT('',(-0.1,-0.67,0.55));
#13374=CARTESIAN_POINT('',(20.,-0.335,0.55));
#13375=CARTESIAN_POINT('Origin',(-0.1,-0.42,0.3));
#13376=CARTESIAN_POINT('',(0.,-0.42,0.3));
#13377=CARTESIAN_POINT('',(-6.93889390390723E-18,-0.24,0.12));
#13378=CARTESIAN_POINT('',(20.,-0.42,0.3));
#13379=CARTESIAN_POINT('',(-0.1,-0.42,0.3));
#13380=CARTESIAN_POINT('',(20.,-0.24,0.12));
#13381=CARTESIAN_POINT('Origin',(-0.1,-0.42,-0.3));
#13382=CARTESIAN_POINT('',(0.,-0.42,-0.3));
#13383=CARTESIAN_POINT('',(0.,-0.42,-0.15));
#13384=CARTESIAN_POINT('',(20.,-0.42,-0.3));
#13385=CARTESIAN_POINT('',(-0.1,-0.42,-0.3));
#13386=CARTESIAN_POINT('',(20.,-0.42,-0.15));
#13387=CARTESIAN_POINT('Origin',(-0.1,-0.67,-0.55));
#13388=CARTESIAN_POINT('',(0.,-0.67,-0.55));
#13389=CARTESIAN_POINT('',(0.,-0.365,-0.245));
#13390=CARTESIAN_POINT('',(20.,-0.67,-0.55));
#13391=CARTESIAN_POINT('',(-0.1,-0.67,-0.55));
#13392=CARTESIAN_POINT('',(20.,-0.365,-0.245));
#13393=CARTESIAN_POINT('Origin',(-0.1,-0.82,-0.55));
#13394=CARTESIAN_POINT('',(0.,-0.82,-0.55));
#13395=CARTESIAN_POINT('',(0.,-0.41,-0.55));
#13396=CARTESIAN_POINT('',(20.,-0.82,-0.55));
#13397=CARTESIAN_POINT('',(-0.1,-0.82,-0.55));
#13398=CARTESIAN_POINT('',(20.,-0.41,-0.55));
#13399=CARTESIAN_POINT('Origin',(-0.1,-0.82,-0.3));
#13400=CARTESIAN_POINT('',(0.,-0.82,-0.3));
#13401=CARTESIAN_POINT('',(0.,-0.82,-0.15));
#13402=CARTESIAN_POINT('',(20.,-0.82,-0.3));
#13403=CARTESIAN_POINT('',(-0.1,-0.82,-0.3));
#13404=CARTESIAN_POINT('',(20.,-0.82,-0.15));
#13405=CARTESIAN_POINT('Origin',(-0.1,-1.05,-0.3));
#13406=CARTESIAN_POINT('',(0.,-1.,-0.3));
#13407=CARTESIAN_POINT('',(0.,-0.525,-0.3));
#13408=CARTESIAN_POINT('',(20.,-1.,-0.3));
#13409=CARTESIAN_POINT('',(-0.05,-1.,-0.3));
#13410=CARTESIAN_POINT('',(20.,-0.525,-0.3));
#13411=CARTESIAN_POINT('Origin',(-0.1,0.3,0.82));
#13412=CARTESIAN_POINT('',(0.,0.3,0.82));
#13413=CARTESIAN_POINT('',(0.,0.3,1.));
#13414=CARTESIAN_POINT('',(0.,0.3,0.41));
#13415=CARTESIAN_POINT('',(20.,0.3,0.82));
#13416=CARTESIAN_POINT('',(-0.1,0.3,0.82));
#13417=CARTESIAN_POINT('',(20.,0.3,1.));
#13418=CARTESIAN_POINT('',(20.,0.3,0.41));
#13419=CARTESIAN_POINT('',(-0.05,0.3,1.));
#13420=CARTESIAN_POINT('Origin',(-0.1,0.55,0.82));
#13421=CARTESIAN_POINT('',(0.,0.55,0.82));
#13422=CARTESIAN_POINT('',(0.,0.275,0.82));
#13423=CARTESIAN_POINT('',(20.,0.55,0.82));
#13424=CARTESIAN_POINT('',(-0.1,0.55,0.82));
#13425=CARTESIAN_POINT('',(20.,0.275,0.82));
#13426=CARTESIAN_POINT('Origin',(-0.1,0.55,0.67));
#13427=CARTESIAN_POINT('',(0.,0.55,0.67));
#13428=CARTESIAN_POINT('',(0.,0.55,0.335));
#13429=CARTESIAN_POINT('',(20.,0.55,0.67));
#13430=CARTESIAN_POINT('',(-0.1,0.55,0.67));
#13431=CARTESIAN_POINT('',(20.,0.55,0.335));
#13432=CARTESIAN_POINT('Origin',(-0.1,0.3,0.42));
#13433=CARTESIAN_POINT('',(0.,0.3,0.42));
#13434=CARTESIAN_POINT('',(6.93889390390723E-18,0.12,0.24));
#13435=CARTESIAN_POINT('',(20.,0.3,0.42));
#13436=CARTESIAN_POINT('',(-0.1,0.3,0.42));
#13437=CARTESIAN_POINT('',(20.,0.12,0.24));
#13438=CARTESIAN_POINT('Origin',(-0.1,-0.3,0.42));
#13439=CARTESIAN_POINT('',(0.,-0.3,0.42));
#13440=CARTESIAN_POINT('',(0.,-0.15,0.42));
#13441=CARTESIAN_POINT('',(20.,-0.3,0.42));
#13442=CARTESIAN_POINT('',(-0.1,-0.3,0.42));
#13443=CARTESIAN_POINT('',(20.,-0.15,0.42));
#13444=CARTESIAN_POINT('Origin',(-0.1,-0.55,0.67));
#13445=CARTESIAN_POINT('',(0.,-0.55,0.67));
#13446=CARTESIAN_POINT('',(6.93889390390723E-18,-0.245,0.365));
#13447=CARTESIAN_POINT('',(20.,-0.55,0.67));
#13448=CARTESIAN_POINT('',(-0.1,-0.55,0.67));
#13449=CARTESIAN_POINT('',(20.,-0.245,0.365));
#13450=CARTESIAN_POINT('Origin',(-0.1,-0.55,0.82));
#13451=CARTESIAN_POINT('',(0.,-0.55,0.82));
#13452=CARTESIAN_POINT('',(0.,-0.55,0.41));
#13453=CARTESIAN_POINT('',(20.,-0.55,0.82));
#13454=CARTESIAN_POINT('',(-0.1,-0.55,0.82));
#13455=CARTESIAN_POINT('',(20.,-0.55,0.41));
#13456=CARTESIAN_POINT('Origin',(-0.1,-0.3,0.82));
#13457=CARTESIAN_POINT('',(0.,-0.3,0.82));
#13458=CARTESIAN_POINT('',(0.,-0.15,0.82));
#13459=CARTESIAN_POINT('',(20.,-0.3,0.82));
#13460=CARTESIAN_POINT('',(-0.1,-0.3,0.82));
#13461=CARTESIAN_POINT('',(20.,-0.15,0.82));
#13462=CARTESIAN_POINT('Origin',(-0.1,-0.3,1.05));
#13463=CARTESIAN_POINT('',(0.,-0.3,1.));
#13464=CARTESIAN_POINT('',(0.,-0.3,0.525));
#13465=CARTESIAN_POINT('',(20.,-0.3,1.));
#13466=CARTESIAN_POINT('',(-0.05,-0.3,1.));
#13467=CARTESIAN_POINT('',(20.,-0.3,0.525));
#13468=CARTESIAN_POINT('Origin',(-0.1,0.,0.));
#13469=CARTESIAN_POINT('',(0.,-2.57175827820944E-17,0.21));
#13470=CARTESIAN_POINT('Origin',(0.,0.,0.));
#13471=CARTESIAN_POINT('',(20.,2.57175827820944E-17,0.21));
#13472=CARTESIAN_POINT('',(-0.1,-2.57175827820944E-17,0.21));
#13473=CARTESIAN_POINT('Origin',(20.,0.,0.));
#13474=CARTESIAN_POINT('Origin',(0.,1.,-1.));
#13475=CARTESIAN_POINT('',(0.,1.,1.));
#13476=CARTESIAN_POINT('',(0.,1.,-1.));
#13477=CARTESIAN_POINT('',(20.,1.,1.));
#13478=CARTESIAN_POINT('',(0.,1.,1.));
#13479=CARTESIAN_POINT('',(20.,1.,-1.));
#13480=CARTESIAN_POINT('Origin',(0.,1.,-1.));
#13481=CARTESIAN_POINT('',(20.,1.,-1.));
#13482=CARTESIAN_POINT('',(20.,1.,-1.));
#13483=CARTESIAN_POINT('',(0.,1.,-1.));
#13484=CARTESIAN_POINT('',(0.,1.,-1.));
#13485=CARTESIAN_POINT('',(0.,1.,-1.));
#13486=CARTESIAN_POINT('Origin',(0.,-1.,-1.));
#13487=CARTESIAN_POINT('',(0.,-1.,-1.));
#13488=CARTESIAN_POINT('',(20.,-1.,-1.));
#13489=CARTESIAN_POINT('Origin',(0.,-1.,-1.));
#13490=CARTESIAN_POINT('',(20.,-1.,-1.));
#13491=CARTESIAN_POINT('',(20.,-1.,-1.));
#13492=CARTESIAN_POINT('',(0.,-1.,-1.));
#13493=CARTESIAN_POINT('',(0.,-1.,-1.));
#13494=CARTESIAN_POINT('',(0.,-1.,-1.));
#13495=CARTESIAN_POINT('Origin',(0.,-1.,1.));
#13496=CARTESIAN_POINT('',(0.,-1.,1.));
#13497=CARTESIAN_POINT('',(20.,-1.,1.));
#13498=CARTESIAN_POINT('Origin',(0.,-1.,1.));
#13499=CARTESIAN_POINT('',(20.,-1.,1.));
#13500=CARTESIAN_POINT('',(20.,-1.,1.));
#13501=CARTESIAN_POINT('',(0.,-1.,1.));
#13502=CARTESIAN_POINT('',(0.,-1.,1.));
#13503=CARTESIAN_POINT('',(0.,-1.,1.));
#13504=CARTESIAN_POINT('Origin',(0.,1.,1.));
#13505=CARTESIAN_POINT('',(0.,1.,1.));
#13506=CARTESIAN_POINT('',(20.,1.,1.));
#13507=CARTESIAN_POINT('Origin',(0.,1.,1.));
#13508=CARTESIAN_POINT('',(20.,1.,1.));
#13509=CARTESIAN_POINT('',(0.,1.,1.));
#13510=CARTESIAN_POINT('Origin',(20.,0.,0.));
#13511=CARTESIAN_POINT('Origin',(0.,0.,0.));
#14428=UNCERTAINTY_MEASURE_WITH_UNIT(LENGTH_MEASURE(0.001),#14479,
'DISTANCE_ACCURACY_VALUE',
'Maximum model space distance between geometric entities at asserted c
onnectivities');
#14446=UNCERTAINTY_MEASURE_WITH_UNIT(LENGTH_MEASURE(0.001),#14479,
'DISTANCE_ACCURACY_VALUE',
'Maximum model space distance between geometric entities at asserted c
onnectivities');
#14460=(
GEOMETRIC_REPRESENTATION_CONTEXT(3)
GLOBAL_UNCERTAINTY_ASSIGNED_CONTEXT((#14428))
GLOBAL_UNIT_ASSIGNED_CONTEXT((#14479,#14481,#14482))
REPRESENTATION_CONTEXT('','3D')
);
#14478=(
GEOMETRIC_REPRESENTATION_CONTEXT(3)
GLOBAL_UNCERTAINTY_ASSIGNED_CONTEXT((#14446))
GLOBAL_UNIT_ASSIGNED_CONTEXT((#14479,#14481,#14482))
REPRESENTATION_CONTEXT('','3D')
);
#14479=(
LENGTH_UNIT()
NAMED_UNIT(*)
SI_UNIT(.CENTI.,.METRE.)
);
#14481=(
NAMED_UNIT(*)
PLANE_ANGLE_UNIT()
SI_UNIT($,.RADIAN.)
);
#14482=(
NAMED_UNIT(*)
SI_UNIT($,.STERADIAN.)
SOLID_ANGLE_UNIT()
);
#14496=SHAPE_DEFINITION_REPRESENTATION(#14527,#14616);
#14527=PRODUCT_DEFINITION_SHAPE('',$,#14648);
#14616=SHAPE_REPRESENTATION('',(#9226),#14460);
#14634=PRODUCT_DEFINITION_CONTEXT('part definition',#14729,'design');
#14648=PRODUCT_DEFINITION('Slotted Extrusion - 20 x 20 x 200 mm',
'Slotted Extrusion - 20 x 20 x 200 mm',#14679,#14634);
#14679=PRODUCT_DEFINITION_FORMATION('',$,#14744);
#14729=APPLICATION_CONTEXT(
'Core Data for Automotive Mechanical Design Process');
#14730=PRODUCT_CONTEXT('part definition',#14729,'mechanical');
#14744=PRODUCT('Slotted Extrusion - 20 x 20 x 200 mm',
'Slotted Extrusion - 20 x 20 x 200 mm',
'Slotted Extrusion - 20 x 20 x 200 mm',(#14730));
#14839=COLOUR_RGB('Off White',0.89,0.88,0.83);
#14840=FILL_AREA_STYLE_COLOUR('',#14839);
#14841=FILL_AREA_STYLE('',(#14840));
#14842=SURFACE_STYLE_FILL_AREA(#14841);
#14843=SURFACE_SIDE_STYLE('',(#14842));
#14844=SURFACE_STYLE_USAGE(.BOTH.,#14843);
#14845=PRESENTATION_STYLE_ASSIGNMENT((#14844));
ENDSEC;
END-ISO-10303-21;
